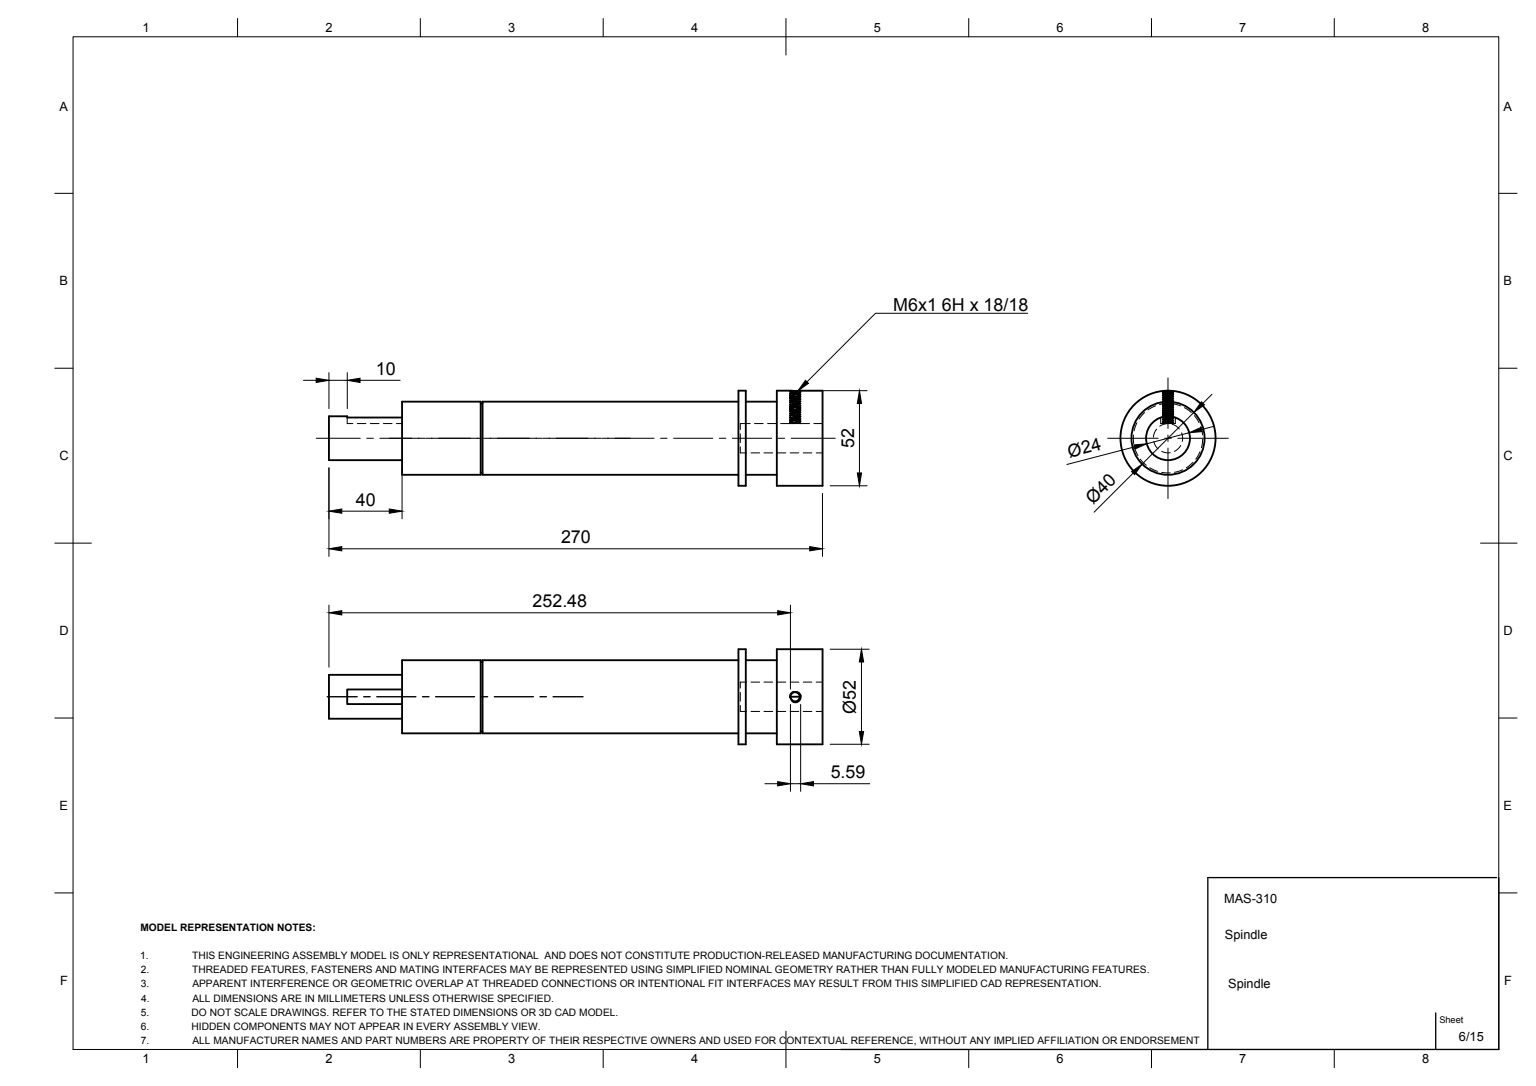
ISO-10303-21;
HEADER;
/* Generated by software containing ST-Developer
 * from STEP Tools, Inc. (www.steptools.com) 
 */

FILE_DESCRIPTION(
/* description */ ('Independent30mm screw-fed quill/spindle unit with16mm straight tool s
ocket, radial set screw, native reusable open ball bearings, retained 
inner/outer race stacks, keyed quill guide and M12x1.75 fine feed. Ext
ernal moving drive and tool not included. Ideal cage orbital links; in
dividual ball spin, force and preload not simulated. No drilling capac
ity, runout, speed, torque, load, life or machine safety rating.'),
/* implementation_level */ '2;1');

FILE_NAME(
/* name */ 'Spindle.step',
/* time_stamp */ '2026-11-08T18:59:42-08:00',
/* author */ (''),
/* organization */ (''),
/* preprocessor_version */ 'ST-DEVELOPER v20.2',
/* originating_system */ 'Autodesk Translation Framework v15.17.0.0',
/* authorisation */ '');

FILE_SCHEMA (('AUTOMOTIVE_DESIGN { 1 0 10303 214 3 1 1 }'));
ENDSEC;

DATA;
#10=MECHANICAL_DESIGN_GEOMETRIC_PRESENTATION_REPRESENTATION('',(#1594),#63898);
#258=B_SPLINE_SURFACE_WITH_KNOTS('',3,3,((#45452,#45453,#45454,#45455,#45456,
#45457,#45458,#45459,#45460,#45461,#45462,#45463,#45464,#45465,#45466,#45467,
#45468,#45469,#45470,#45471,#45472,#45473,#45474,#45475,#45476,#45477,#45478,
#45479,#45480,#45481,#45482,#45483,#45484,#45485,#45486,#45487,#45488,#45489,
#45490,#45491,#45492,#45493,#45494,#45495,#45496,#45497,#45498,#45499,#45500,
#45501,#45502,#45503,#45504,#45505,#45506,#45507,#45508,#45509,#45510,#45511,
#45512,#45513,#45514,#45515,#45516,#45517,#45518,#45519,#45520,#45521,#45522,
#45523,#45524,#45525,#45526,#45527,#45528,#45529,#45530,#45531,#45532,#45533,
#45534,#45535,#45536,#45537,#45538,#45539,#45540,#45541,#45542,#45543,#45544,
#45545,#45546,#45547,#45548,#45549,#45550,#45551,#45552,#45553,#45554,#45555,
#45556,#45557,#45558,#45559,#45560,#45561,#45562,#45563,#45564,#45565,#45566,
#45567,#45568,#45569),(#45570,#45571,#45572,#45573,#45574,#45575,#45576,
#45577,#45578,#45579,#45580,#45581,#45582,#45583,#45584,#45585,#45586,#45587,
#45588,#45589,#45590,#45591,#45592,#45593,#45594,#45595,#45596,#45597,#45598,
#45599,#45600,#45601,#45602,#45603,#45604,#45605,#45606,#45607,#45608,#45609,
#45610,#45611,#45612,#45613,#45614,#45615,#45616,#45617,#45618,#45619,#45620,
#45621,#45622,#45623,#45624,#45625,#45626,#45627,#45628,#45629,#45630,#45631,
#45632,#45633,#45634,#45635,#45636,#45637,#45638,#45639,#45640,#45641,#45642,
#45643,#45644,#45645,#45646,#45647,#45648,#45649,#45650,#45651,#45652,#45653,
#45654,#45655,#45656,#45657,#45658,#45659,#45660,#45661,#45662,#45663,#45664,
#45665,#45666,#45667,#45668,#45669,#45670,#45671,#45672,#45673,#45674,#45675,
#45676,#45677,#45678,#45679,#45680,#45681,#45682,#45683,#45684,#45685,#45686,
#45687),(#45688,#45689,#45690,#45691,#45692,#45693,#45694,#45695,#45696,
#45697,#45698,#45699,#45700,#45701,#45702,#45703,#45704,#45705,#45706,#45707,
#45708,#45709,#45710,#45711,#45712,#45713,#45714,#45715,#45716,#45717,#45718,
#45719,#45720,#45721,#45722,#45723,#45724,#45725,#45726,#45727,#45728,#45729,
#45730,#45731,#45732,#45733,#45734,#45735,#45736,#45737,#45738,#45739,#45740,
#45741,#45742,#45743,#45744,#45745,#45746,#45747,#45748,#45749,#45750,#45751,
#45752,#45753,#45754,#45755,#45756,#45757,#45758,#45759,#45760,#45761,#45762,
#45763,#45764,#45765,#45766,#45767,#45768,#45769,#45770,#45771,#45772,#45773,
#45774,#45775,#45776,#45777,#45778,#45779,#45780,#45781,#45782,#45783,#45784,
#45785,#45786,#45787,#45788,#45789,#45790,#45791,#45792,#45793,#45794,#45795,
#45796,#45797,#45798,#45799,#45800,#45801,#45802,#45803,#45804,#45805),
(#45806,#45807,#45808,#45809,#45810,#45811,#45812,#45813,#45814,#45815,
#45816,#45817,#45818,#45819,#45820,#45821,#45822,#45823,#45824,#45825,#45826,
#45827,#45828,#45829,#45830,#45831,#45832,#45833,#45834,#45835,#45836,#45837,
#45838,#45839,#45840,#45841,#45842,#45843,#45844,#45845,#45846,#45847,#45848,
#45849,#45850,#45851,#45852,#45853,#45854,#45855,#45856,#45857,#45858,#45859,
#45860,#45861,#45862,#45863,#45864,#45865,#45866,#45867,#45868,#45869,#45870,
#45871,#45872,#45873,#45874,#45875,#45876,#45877,#45878,#45879,#45880,#45881,
#45882,#45883,#45884,#45885,#45886,#45887,#45888,#45889,#45890,#45891,#45892,
#45893,#45894,#45895,#45896,#45897,#45898,#45899,#45900,#45901,#45902,#45903,
#45904,#45905,#45906,#45907,#45908,#45909,#45910,#45911,#45912,#45913,#45914,
#45915,#45916,#45917,#45918,#45919,#45920,#45921,#45922,#45923)),
 .UNSPECIFIED.,.F.,.F.,.F.,(4,4),(4,1,1,1,1,1,1,1,1,1,1,1,1,1,1,1,1,1,1,
1,1,1,1,1,1,1,1,1,1,1,1,1,1,1,1,1,1,1,1,1,1,1,1,1,1,1,1,1,1,1,1,1,1,1,1,
1,1,1,1,1,1,1,1,1,1,1,1,1,1,1,1,1,1,1,1,1,1,1,1,1,1,1,1,1,1,1,1,1,1,1,1,
1,1,1,1,1,1,1,1,1,1,1,1,1,1,1,1,1,1,1,1,1,1,1,1,4),(0.,0.0642013499338863),
(12.6240367263184,13.6183778789988,14.6127190316793,15.6070601843597,16.6014013370402,
17.5957424897206,18.590083642401,19.5844247950815,20.5787659477619,21.5731071004423,
22.5674482531228,23.5617894058032,24.5561305584837,25.5504717111641,26.5448128638445,
27.539154016525,28.5334951692054,29.5278363218858,30.5221774745663,31.5165186272467,
32.5108597799272,33.5052009326076,34.499542085288,35.4938832379685,36.4882243906489,
37.4825655433293,38.4769066960098,39.4712478486902,40.4655890013707,41.4599301540511,
42.4542713067315,43.448612459412,44.4429536120924,45.4372947647728,46.4316359174533,
47.4259770701337,48.4203182228142,49.4146593754946,50.409000528175,51.4033416808555,
52.3976828335359,53.3920239862163,54.3863651388968,55.3807062915772,56.3750474442577,
57.3693885969381,58.3637297496185,59.358070902299,60.3524120549794,61.3467532076598,
62.3410943603403,63.3354355130207,64.3297766657012,65.3241178183816,66.318458971062,
67.3128001237425,68.3071412764229,69.3014824291033,70.2958235817838,71.2901647344642,
72.2845058871447,73.2788470398251,74.2731881925055,75.267529345186,76.2618704978664,
77.2562116505468,78.2505528032273,79.2448939559077,80.2392351085882,81.2335762612686,
82.227917413949,83.2222585666295,84.2165997193099,85.2109408719903,86.2052820246708,
87.1996231773512,88.1939643300317,89.1883054827121,90.1826466353925,91.176987788073,
92.1713289407534,93.1656700934338,94.1600112461143,95.1543523987947,96.1486935514752,
97.1430347041556,98.137375856836,99.1317170095165,100.126058162197,101.120399314877,
102.114740467558,103.109081620238,104.103422772919,105.097763925599,106.09210507828,
107.08644623096,108.08078738364,109.075128536321,110.069469689001,111.063810841682,
112.058151994362,113.052493147043,114.046834299723,115.041175452403,116.035516605084,
117.029857757764,118.024198910445,119.018540063125,120.012881215806,121.007222368486,
122.001563521167,122.995904673847,123.990245826527,124.984586979208,125.978928131888,
126.973269284569),.UNSPECIFIED.);
#259=B_SPLINE_SURFACE_WITH_KNOTS('',3,3,((#46071,#46072,#46073,#46074,#46075,
#46076,#46077,#46078,#46079,#46080,#46081,#46082,#46083,#46084,#46085,#46086,
#46087,#46088,#46089,#46090,#46091,#46092,#46093,#46094,#46095,#46096,#46097,
#46098,#46099,#46100,#46101,#46102,#46103,#46104,#46105,#46106,#46107,#46108,
#46109,#46110,#46111,#46112,#46113,#46114,#46115,#46116,#46117,#46118,#46119,
#46120,#46121,#46122,#46123,#46124,#46125,#46126,#46127,#46128,#46129,#46130,
#46131,#46132,#46133,#46134,#46135,#46136,#46137,#46138,#46139,#46140,#46141,
#46142,#46143,#46144,#46145,#46146,#46147,#46148,#46149,#46150,#46151,#46152,
#46153,#46154,#46155,#46156,#46157,#46158,#46159,#46160,#46161,#46162,#46163,
#46164,#46165,#46166,#46167,#46168,#46169,#46170,#46171,#46172,#46173,#46174,
#46175,#46176,#46177,#46178,#46179,#46180,#46181,#46182,#46183,#46184,#46185,
#46186,#46187,#46188),(#46189,#46190,#46191,#46192,#46193,#46194,#46195,
#46196,#46197,#46198,#46199,#46200,#46201,#46202,#46203,#46204,#46205,#46206,
#46207,#46208,#46209,#46210,#46211,#46212,#46213,#46214,#46215,#46216,#46217,
#46218,#46219,#46220,#46221,#46222,#46223,#46224,#46225,#46226,#46227,#46228,
#46229,#46230,#46231,#46232,#46233,#46234,#46235,#46236,#46237,#46238,#46239,
#46240,#46241,#46242,#46243,#46244,#46245,#46246,#46247,#46248,#46249,#46250,
#46251,#46252,#46253,#46254,#46255,#46256,#46257,#46258,#46259,#46260,#46261,
#46262,#46263,#46264,#46265,#46266,#46267,#46268,#46269,#46270,#46271,#46272,
#46273,#46274,#46275,#46276,#46277,#46278,#46279,#46280,#46281,#46282,#46283,
#46284,#46285,#46286,#46287,#46288,#46289,#46290,#46291,#46292,#46293,#46294,
#46295,#46296,#46297,#46298,#46299,#46300,#46301,#46302,#46303,#46304,#46305,
#46306),(#46307,#46308,#46309,#46310,#46311,#46312,#46313,#46314,#46315,
#46316,#46317,#46318,#46319,#46320,#46321,#46322,#46323,#46324,#46325,#46326,
#46327,#46328,#46329,#46330,#46331,#46332,#46333,#46334,#46335,#46336,#46337,
#46338,#46339,#46340,#46341,#46342,#46343,#46344,#46345,#46346,#46347,#46348,
#46349,#46350,#46351,#46352,#46353,#46354,#46355,#46356,#46357,#46358,#46359,
#46360,#46361,#46362,#46363,#46364,#46365,#46366,#46367,#46368,#46369,#46370,
#46371,#46372,#46373,#46374,#46375,#46376,#46377,#46378,#46379,#46380,#46381,
#46382,#46383,#46384,#46385,#46386,#46387,#46388,#46389,#46390,#46391,#46392,
#46393,#46394,#46395,#46396,#46397,#46398,#46399,#46400,#46401,#46402,#46403,
#46404,#46405,#46406,#46407,#46408,#46409,#46410,#46411,#46412,#46413,#46414,
#46415,#46416,#46417,#46418,#46419,#46420,#46421,#46422,#46423,#46424),
(#46425,#46426,#46427,#46428,#46429,#46430,#46431,#46432,#46433,#46434,
#46435,#46436,#46437,#46438,#46439,#46440,#46441,#46442,#46443,#46444,#46445,
#46446,#46447,#46448,#46449,#46450,#46451,#46452,#46453,#46454,#46455,#46456,
#46457,#46458,#46459,#46460,#46461,#46462,#46463,#46464,#46465,#46466,#46467,
#46468,#46469,#46470,#46471,#46472,#46473,#46474,#46475,#46476,#46477,#46478,
#46479,#46480,#46481,#46482,#46483,#46484,#46485,#46486,#46487,#46488,#46489,
#46490,#46491,#46492,#46493,#46494,#46495,#46496,#46497,#46498,#46499,#46500,
#46501,#46502,#46503,#46504,#46505,#46506,#46507,#46508,#46509,#46510,#46511,
#46512,#46513,#46514,#46515,#46516,#46517,#46518,#46519,#46520,#46521,#46522,
#46523,#46524,#46525,#46526,#46527,#46528,#46529,#46530,#46531,#46532,#46533,
#46534,#46535,#46536,#46537,#46538,#46539,#46540,#46541,#46542)),
 .UNSPECIFIED.,.F.,.F.,.F.,(4,4),(4,1,1,1,1,1,1,1,1,1,1,1,1,1,1,1,1,1,1,
1,1,1,1,1,1,1,1,1,1,1,1,1,1,1,1,1,1,1,1,1,1,1,1,1,1,1,1,1,1,1,1,1,1,1,1,
1,1,1,1,1,1,1,1,1,1,1,1,1,1,1,1,1,1,1,1,1,1,1,1,1,1,1,1,1,1,1,1,1,1,1,1,
1,1,1,1,1,1,1,1,1,1,1,1,1,1,1,1,1,1,1,1,1,1,1,1,4),(0.,0.0642013499338863),
(15.4901713080479,16.481671388406,17.4731714687642,18.4646715491223,19.4561716294804,
20.4476717098386,21.4391717901967,22.4306718705548,23.4221719509129,24.4136720312711,
25.4051721116292,26.3966721919873,27.3881722723455,28.3796723527036,29.3711724330617,
30.3626725134198,31.354172593778,32.3456726741361,33.3371727544942,34.3286728348524,
35.3201729152105,36.3116729955686,37.3031730759268,38.2946731562849,39.286173236643,
40.2776733170011,41.2691733973593,42.2606734777174,43.2521735580755,44.2436736384336,
45.2351737187918,46.2266737991499,47.218173879508,48.2096739598662,49.2011740402243,
50.1926741205824,51.1841742009405,52.1756742812987,53.1671743616568,54.1586744420149,
55.1501745223731,56.1416746027312,57.1331746830893,58.1246747634475,59.1161748438056,
60.1076749241637,61.0991750045218,62.09067508488,63.0821751652381,64.0736752455962,
65.0651753259544,66.0566754063125,67.0481754866706,68.0396755670287,69.0311756473869,
70.022675727745,71.0141758081031,72.0056758884613,72.9971759688194,73.9886760491775,
74.9801761295356,75.9716762098938,76.9631762902519,77.95467637061,78.9461764509682,
79.9376765313263,80.9291766116844,81.9206766920425,82.9121767724007,83.9036768527588,
84.8951769331169,85.8866770134751,86.8781770938332,87.8696771741913,88.8611772545494,
89.8526773349076,90.8441774152657,91.8356774956238,92.827177575982,93.8186776563401,
94.8101777366982,95.8016778170563,96.7931778974145,97.7846779777726,98.7761780581307,
99.7676781384889,100.759178218847,101.750678299205,102.742178379563,103.733678459921,
104.72517854028,105.716678620638,106.708178700996,107.699678781354,108.691178861712,
109.68267894207,110.674179022428,111.665679102786,112.657179183145,113.648679263503,
114.640179343861,115.631679424219,116.623179504577,117.614679584935,118.606179665293,
119.597679745651,120.58917982601,121.580679906368,122.572179986726,123.563680067084,
124.555180147442,125.5466802278,126.538180308158,127.529680388516,128.521180468875,
129.512680549233),.UNSPECIFIED.);
#957=B_SPLINE_CURVE_WITH_KNOTS('',3,(#44085,#44086,#44087,#44088),
 .UNSPECIFIED.,.F.,.F.,(4,4),(114.40689867021,115.114280422261),
 .UNSPECIFIED.);
#958=B_SPLINE_CURVE_WITH_KNOTS('',3,(#44093,#44094,#44095,#44096,#44097,
#44098,#44099,#44100,#44101,#44102),.UNSPECIFIED.,.F.,.F.,(4,3,3,4),(-113.097335529233,
-112.13125696422,-111.136915811539,-110.663124627694),.UNSPECIFIED.);
#959=B_SPLINE_CURVE_WITH_KNOTS('',3,(#44107,#44108,#44109,#44110,#44111,
#44112,#44113,#44114,#44115,#44116,#44117,#44118,#44119,#44120,#44121,#44122,
#44123,#44124,#44125,#44126,#44127,#44128,#44129,#44130,#44131),
 .UNSPECIFIED.,.F.,.F.,(4,3,3,3,3,3,3,3,4),(108.12371336303,108.173779859754,
109.165279940112,110.15678002047,111.148280100828,112.139780181187,113.131280261545,
114.122780341903,114.40689867021),.UNSPECIFIED.);
#960=B_SPLINE_CURVE_WITH_KNOTS('',3,(#44132,#44133,#44134,#44135,#44136,
#44137,#44138,#44139,#44140,#44141,#44142,#44143,#44144,#44145,#44146,#44147,
#44148,#44149,#44150,#44151,#44152,#44153),.UNSPECIFIED.,.F.,.F.,(4,3,3,
3,3,3,3,4),(-110.663124627694,-110.142574658859,-109.148233506178,-108.153892353498,
-107.159551200817,-106.165210048137,-105.170868895457,-104.379939320515),
 .UNSPECIFIED.);
#961=B_SPLINE_CURVE_WITH_KNOTS('',3,(#44158,#44159,#44160,#44161,#44162,
#44163,#44164,#44165,#44166,#44167,#44168,#44169,#44170,#44171,#44172,#44173,
#44174,#44175,#44176,#44177,#44178,#44179),.UNSPECIFIED.,.F.,.F.,(4,3,3,
3,3,3,3,4),(101.84052805585,102.224779377605,103.216279457963,104.207779538322,
105.19927961868,106.190779699038,107.182279779396,108.12371336303),
 .UNSPECIFIED.);
#962=B_SPLINE_CURVE_WITH_KNOTS('',3,(#44180,#44181,#44182,#44183,#44184,
#44185,#44186,#44187,#44188,#44189,#44190,#44191,#44192,#44193,#44194,#44195,
#44196,#44197,#44198,#44199,#44200,#44201,#44202,#44203,#44204),
 .UNSPECIFIED.,.F.,.F.,(4,3,3,3,3,3,3,3,4),(-104.379939320515,-104.176527742776,
-103.182186590096,-102.187845437415,-101.193504284735,-100.199163132054,
-99.204821979374,-98.2104808266935,-98.096754013335),.UNSPECIFIED.);
#963=B_SPLINE_CURVE_WITH_KNOTS('',3,(#44209,#44210,#44211,#44212,#44213,
#44214,#44215,#44216,#44217,#44218,#44219,#44220,#44221,#44222,#44223,#44224,
#44225,#44226,#44227,#44228,#44229,#44230),.UNSPECIFIED.,.F.,.F.,(4,3,3,
3,3,3,3,4),(95.5573427486709,96.2757788954565,97.2672789758147,98.2587790561728,
99.2502791365309,100.241779216889,101.233279297247,101.84052805585),
 .UNSPECIFIED.);
#964=B_SPLINE_CURVE_WITH_KNOTS('',3,(#44231,#44232,#44233,#44234,#44235,
#44236,#44237,#44238,#44239,#44240,#44241,#44242,#44243,#44244,#44245,#44246,
#44247,#44248,#44249,#44250,#44251,#44252),.UNSPECIFIED.,.F.,.F.,(4,3,3,
3,3,3,3,4),(-98.096754013335,-97.2161396740131,-96.2217985213327,-95.2274573686523,
-94.2331162159718,-93.2387750632914,-92.2444339106109,-91.8135687061554),
 .UNSPECIFIED.);
#965=B_SPLINE_CURVE_WITH_KNOTS('',3,(#44257,#44258,#44259,#44260,#44261,
#44262,#44263,#44264,#44265,#44266,#44267,#44268,#44269,#44270,#44271,#44272,
#44273,#44274,#44275,#44276,#44277,#44278,#44279,#44280,#44281),
 .UNSPECIFIED.,.F.,.F.,(4,3,3,3,3,3,3,3,4),(89.2741574414913,89.3352783329496,
90.3267784133077,91.3182784936659,92.309778574024,93.3012786543821,94.2927787347403,
95.2842788150984,95.5573427486709),.UNSPECIFIED.);
#966=B_SPLINE_CURVE_WITH_KNOTS('',3,(#44282,#44283,#44284,#44285,#44286,
#44287,#44288,#44289,#44290,#44291,#44292,#44293,#44294,#44295,#44296,#44297,
#44298,#44299,#44300,#44301,#44302,#44303),.UNSPECIFIED.,.F.,.F.,(4,3,3,
3,3,3,3,4),(-91.8135687061554,-91.2500927579305,-90.2557516052501,-89.2614104525696,
-88.2670692998892,-87.2727281472088,-86.2783869945283,-85.5303833989758),
 .UNSPECIFIED.);
#967=B_SPLINE_CURVE_WITH_KNOTS('',3,(#44308,#44309,#44310,#44311,#44312,
#44313,#44314,#44315,#44316,#44317,#44318,#44319,#44320,#44321,#44322,#44323,
#44324,#44325,#44326,#44327,#44328,#44329),.UNSPECIFIED.,.F.,.F.,(4,3,3,
3,3,3,3,4),(82.9909721343117,83.3862778508009,84.377777931159,85.3692780115171,
86.3607780918753,87.3522781722334,88.3437782525915,89.2741574414913),
 .UNSPECIFIED.);
#968=B_SPLINE_CURVE_WITH_KNOTS('',3,(#44330,#44331,#44332,#44333,#44334,
#44335,#44336,#44337,#44338,#44339,#44340,#44341,#44342,#44343,#44344,#44345,
#44346,#44347,#44348,#44349,#44350,#44351,#44352,#44353,#44354),
 .UNSPECIFIED.,.F.,.F.,(4,3,3,3,3,3,3,3,4),(-85.5303833989758,-85.2840458418479,
-84.2897046891674,-83.295363536487,-82.3010223838066,-81.3066812311261,
-80.3123400784457,-79.3179989257652,-79.2471980917962),.UNSPECIFIED.);
#969=B_SPLINE_CURVE_WITH_KNOTS('',3,(#44359,#44360,#44361,#44362,#44363,
#44364,#44365,#44366,#44367,#44368,#44369,#44370,#44371,#44372,#44373,#44374,
#44375,#44376,#44377,#44378,#44379,#44380),.UNSPECIFIED.,.F.,.F.,(4,3,3,
3,3,3,3,4),(76.7077868271321,77.4372773686521,78.4287774490102,79.4202775293683,
80.4117776097265,81.4032776900846,82.3947777704427,82.9909721343117),
 .UNSPECIFIED.);
#970=B_SPLINE_CURVE_WITH_KNOTS('',3,(#44381,#44382,#44383,#44384,#44385,
#44386,#44387,#44388,#44389,#44390,#44391,#44392,#44393,#44394,#44395,#44396,
#44397,#44398,#44399,#44400,#44401,#44402),.UNSPECIFIED.,.F.,.F.,(4,3,3,
3,3,3,3,4),(-79.2471980917962,-78.3236577730848,-77.3293166204044,-76.3349754677239,
-75.3406343150435,-74.3462931623631,-73.3519520096826,-72.9640127846166),
 .UNSPECIFIED.);
#971=B_SPLINE_CURVE_WITH_KNOTS('',3,(#44407,#44408,#44409,#44410,#44411,
#44412,#44413,#44414,#44415,#44416,#44417,#44418,#44419,#44420,#44421,#44422,
#44423,#44424,#44425,#44426,#44427,#44428,#44429,#44430,#44431),
 .UNSPECIFIED.,.F.,.F.,(4,3,3,3,3,3,3,3,4),(70.4246015199525,70.4967768061452,
71.4882768865033,72.4797769668614,73.4712770472196,74.4627771275777,75.4542772079358,
76.445777288294,76.7077868271321),.UNSPECIFIED.);
#972=B_SPLINE_CURVE_WITH_KNOTS('',3,(#44432,#44433,#44434,#44435,#44436,
#44437,#44438,#44439,#44440,#44441,#44442,#44443,#44444,#44445,#44446,#44447,
#44448,#44449,#44450,#44451,#44452,#44453),.UNSPECIFIED.,.F.,.F.,(4,3,3,
3,3,3,3,4),(-72.9640127846166,-72.3576108570022,-71.3632697043217,-70.3689285516413,
-69.3745873989609,-68.3802462462804,-67.3859050936,-66.680827477437),
 .UNSPECIFIED.);
#973=B_SPLINE_CURVE_WITH_KNOTS('',3,(#44458,#44459,#44460,#44461,#44462,
#44463,#44464,#44465,#44466,#44467,#44468,#44469,#44470,#44471,#44472,#44473,
#44474,#44475,#44476,#44477,#44478,#44479),.UNSPECIFIED.,.F.,.F.,(4,3,3,
3,3,3,3,4),(64.1414162127729,64.5477763239964,65.5392764043545,66.5307764847127,
67.5222765650708,68.5137766454289,69.5052767257871,70.4246015199525),
 .UNSPECIFIED.);
#974=B_SPLINE_CURVE_WITH_KNOTS('',3,(#44480,#44481,#44482,#44483,#44484,
#44485,#44486,#44487,#44488,#44489,#44490,#44491,#44492,#44493,#44494,#44495,
#44496,#44497,#44498,#44499,#44500,#44501,#44502,#44503,#44504),
 .UNSPECIFIED.,.F.,.F.,(4,3,3,3,3,3,3,3,4),(-66.680827477437,-66.3915639409195,
-65.3972227882391,-64.4028816355587,-63.4085404828782,-62.4141993301978,
-61.4198581775174,-60.4255170248369,-60.3976421702574),.UNSPECIFIED.);
#975=B_SPLINE_CURVE_WITH_KNOTS('',3,(#44509,#44510,#44511,#44512,#44513,
#44514,#44515,#44516,#44517,#44518,#44519,#44520,#44521,#44522,#44523,#44524,
#44525,#44526,#44527,#44528,#44529,#44530),.UNSPECIFIED.,.F.,.F.,(4,3,3,
3,3,3,3,4),(57.8582309055933,58.5987758418476,59.5902759222058,60.5817760025639,
61.573276082922,62.5647761632802,63.5562762436383,64.1414162127729),
 .UNSPECIFIED.);
#976=B_SPLINE_CURVE_WITH_KNOTS('',3,(#44531,#44532,#44533,#44534,#44535,
#44536,#44537,#44538,#44539,#44540,#44541,#44542,#44543,#44544,#44545,#44546,
#44547,#44548,#44549,#44550,#44551,#44552),.UNSPECIFIED.,.F.,.F.,(4,3,3,
3,3,3,3,4),(-60.3976421702574,-59.4311758721565,-58.4368347194761,-57.4424935667956,
-56.4481524141152,-55.4538112614347,-54.4594701087543,-54.1144568630778),
 .UNSPECIFIED.);
#977=B_SPLINE_CURVE_WITH_KNOTS('',3,(#44557,#44558,#44559,#44560,#44561,
#44562,#44563,#44564,#44565,#44566,#44567,#44568,#44569,#44570,#44571,#44572,
#44573,#44574,#44575,#44576,#44577,#44578,#44579,#44580,#44581),
 .UNSPECIFIED.,.F.,.F.,(4,3,3,3,3,3,3,3,4),(51.5750455984137,51.6582752793407,
52.6497753596989,53.641275440057,54.6327755204151,55.6242756007733,56.6157756811314,
57.6072757614895,57.8582309055933),.UNSPECIFIED.);
#978=B_SPLINE_CURVE_WITH_KNOTS('',3,(#44582,#44583,#44584,#44585,#44586,
#44587,#44588,#44589,#44590,#44591,#44592,#44593,#44594,#44595,#44596,#44597,
#44598,#44599,#44600,#44601,#44602,#44603),.UNSPECIFIED.,.F.,.F.,(4,3,3,
3,3,3,3,4),(-54.1144568630778,-53.4651289560739,-52.4707878033934,-51.476446650713,
-50.4821054980325,-49.4877643453521,-48.4934231926717,-47.8312715558982),
 .UNSPECIFIED.);
#979=B_SPLINE_CURVE_WITH_KNOTS('',3,(#44608,#44609,#44610,#44611,#44612,
#44613,#44614,#44615,#44616,#44617,#44618,#44619,#44620,#44621,#44622,#44623,
#44624,#44625,#44626,#44627,#44628,#44629),.UNSPECIFIED.,.F.,.F.,(4,3,3,
3,3,3,3,4),(45.2918602912341,45.709274797192,46.7007748775501,47.6922749579082,
48.6837750382664,49.6752751186245,50.6667751989826,51.5750455984137),
 .UNSPECIFIED.);
#980=B_SPLINE_CURVE_WITH_KNOTS('',3,(#44630,#44631,#44632,#44633,#44634,
#44635,#44636,#44637,#44638,#44639,#44640,#44641,#44642,#44643,#44644,#44645,
#44646,#44647,#44648,#44649,#44650,#44651),.UNSPECIFIED.,.F.,.F.,(4,3,3,
3,3,3,3,4),(-47.8312715558982,-47.4990820399912,-46.5047408873108,-45.5103997346304,
-44.5160585819499,-43.5217174292695,-42.5273762765891,-41.5480862487186),
 .UNSPECIFIED.);
#981=B_SPLINE_CURVE_WITH_KNOTS('',3,(#44656,#44657,#44658,#44659,#44660,
#44661,#44662,#44663,#44664,#44665,#44666,#44667,#44668,#44669,#44670,#44671,
#44672,#44673,#44674,#44675,#44676,#44677),.UNSPECIFIED.,.F.,.F.,(4,3,3,
3,3,3,3,4),(39.0086749840545,39.7602743150432,40.7517743954013,41.7432744757595,
42.7347745561176,43.7262746364757,44.7177747168338,45.2918602912341),
 .UNSPECIFIED.);
#982=B_SPLINE_CURVE_WITH_KNOTS('',3,(#44678,#44679,#44680,#44681,#44682,
#44683,#44684,#44685,#44686,#44687,#44688,#44689,#44690,#44691,#44692,#44693,
#44694,#44695,#44696,#44697,#44698,#44699,#44700,#44701,#44702),
 .UNSPECIFIED.,.F.,.F.,(4,3,3,3,3,3,3,3,4),(-41.5480862487186,-41.5330351239086,
-40.5386939712282,-39.5443528185478,-38.5500116658673,-37.5556705131869,
-36.5613293605064,-35.566988207826,-35.264900941539),.UNSPECIFIED.);
#983=B_SPLINE_CURVE_WITH_KNOTS('',3,(#44707,#44708,#44709,#44710,#44711,
#44712,#44713,#44714,#44715,#44716,#44717,#44718,#44719,#44720,#44721,#44722,
#44723,#44724,#44725,#44726,#44727,#44728,#44729,#44730,#44731),
 .UNSPECIFIED.,.F.,.F.,(4,3,3,3,3,3,3,3,4),(32.725489676875,32.8197737525363,
33.8112738328944,34.8027739132525,35.7942739936107,36.7857740739688,37.7772741543269,
38.7687742346851,39.0086749840545),.UNSPECIFIED.);
#984=B_SPLINE_CURVE_WITH_KNOTS('',3,(#44732,#44733,#44734,#44735,#44736,
#44737,#44738,#44739,#44740,#44741,#44742,#44743,#44744,#44745,#44746,#44747,
#44748,#44749,#44750,#44751,#44752,#44753),.UNSPECIFIED.,.F.,.F.,(4,3,3,
3,3,3,3,4),(-35.264900941539,-34.5726470551456,-33.5783059024651,-32.5839647497847,
-31.5896235971042,-30.5952824444238,-29.6009412917434,-28.9817156343595),
 .UNSPECIFIED.);
#985=B_SPLINE_CURVE_WITH_KNOTS('',3,(#44758,#44759,#44760,#44761,#44762,
#44763,#44764,#44765,#44766,#44767,#44768,#44769,#44770,#44771,#44772,#44773,
#44774,#44775,#44776,#44777,#44778,#44779),.UNSPECIFIED.,.F.,.F.,(4,3,3,
3,3,3,3,4),(26.4423043696954,26.8707732703875,27.8622733507456,28.8537734311038,
29.8452735114619,30.83677359182,31.8282736721782,32.725489676875),
 .UNSPECIFIED.);
#986=B_SPLINE_CURVE_WITH_KNOTS('',3,(#44780,#44781,#44782,#44783,#44784,
#44785,#44786,#44787,#44788,#44789,#44790,#44791,#44792,#44793,#44794,#44795,
#44796,#44797,#44798,#44799,#44800,#44801),.UNSPECIFIED.,.F.,.F.,(4,3,3,
3,3,3,3,4),(-28.9817156343595,-28.6066001390629,-27.6122589863825,-26.6179178337021,
-25.6235766810216,-24.6292355283412,-23.6348943756607,-22.6985303271799),
 .UNSPECIFIED.);
#987=B_SPLINE_CURVE_WITH_KNOTS('',3,(#44806,#44807,#44808,#44809,#44810,
#44811,#44812,#44813,#44814,#44815,#44816,#44817,#44818,#44819,#44820,#44821,
#44822,#44823,#44824,#44825,#44826,#44827),.UNSPECIFIED.,.F.,.F.,(4,3,3,
3,3,3,3,4),(20.1591190625158,20.9217727882387,21.9132728685969,22.904772948955,
23.8962730293131,24.8877731096713,25.8792731900294,26.4423043696954),
 .UNSPECIFIED.);
#988=B_SPLINE_CURVE_WITH_KNOTS('',3,(#44828,#44829,#44830,#44831,#44832,
#44833,#44834,#44835,#44836,#44837,#44838,#44839,#44840,#44841,#44842,#44843,
#44844,#44845,#44846,#44847,#44848,#44849,#44850,#44851,#44852),
 .UNSPECIFIED.,.F.,.F.,(4,3,3,3,3,3,3,3,4),(-22.6985303271799,-22.6405532229803,
-21.6462120702999,-20.6518709176194,-19.657529764939,-18.6631886122585,
-17.6688474595781,-16.6745063068977,-16.4153450200003),.UNSPECIFIED.);
#989=B_SPLINE_CURVE_WITH_KNOTS('',3,(#44857,#44858,#44859,#44860,#44861,
#44862,#44863,#44864,#44865,#44866,#44867,#44868,#44869,#44870,#44871,#44872,
#44873,#44874,#44875,#44876,#44877,#44878,#44879,#44880,#44881),
 .UNSPECIFIED.,.F.,.F.,(4,3,3,3,3,3,3,3,4),(13.8759337553362,13.9812722257318,
14.97277230609,15.9642723864481,16.9557724668062,17.9472725471644,18.9387726275225,
19.9302727078806,20.1591190625158),.UNSPECIFIED.);
#990=B_SPLINE_CURVE_WITH_KNOTS('',3,(#44882,#44883,#44884,#44885,#44886,
#44887,#44888,#44889,#44890,#44891,#44892,#44893,#44894,#44895,#44896,#44897,
#44898,#44899,#44900,#44901,#44902,#44903),.UNSPECIFIED.,.F.,.F.,(4,3,3,
3,3,3,3,4),(-16.4153450200003,-15.6801651542172,-14.6858240015368,-13.6914828488564,
-12.6971416961759,-11.7028005434955,-10.708459390815,-10.1321597128207),
 .UNSPECIFIED.);
#991=B_SPLINE_CURVE_WITH_KNOTS('',3,(#44909,#44910,#44911,#44912,#44913,
#44914,#44915,#44916,#44917,#44918,#44919,#44920,#44921),.UNSPECIFIED.,
 .F.,.F.,(4,3,3,3,4),(-3.84897440564112,-3.74807132205199,-2.75373016937155,
-1.75938901669111,-0.765047864010683),.UNSPECIFIED.);
#992=B_SPLINE_CURVE_WITH_KNOTS('',3,(#44923,#44924,#44925,#44926,#44927,
#44928,#44929,#44930,#44931,#44932,#44933,#44934,#44935,#44936,#44937,#44938),
 .UNSPECIFIED.,.F.,.F.,(4,2,2,2,2,2,2,4),(0.232635770676731,0.284684236160853,
0.379578792383291,0.47447334860573,0.569367904828168,0.664262744797375,
0.759157584766583,0.773538308589687),.UNSPECIFIED.);
#993=B_SPLINE_CURVE_WITH_KNOTS('',3,(#44939,#44940,#44941,#44942,#44943,
#44944,#44945,#44946,#44947,#44948,#44949,#44950,#44951,#44952,#44953,#44954,
#44955,#44956,#44957),.UNSPECIFIED.,.F.,.F.,(4,3,3,3,3,3,4),(2.26925352322945,
3.07477134179243,4.06627142215055,5.05777150250868,6.04927158286681,7.04077166322494,
7.59274844815659),.UNSPECIFIED.);
#994=B_SPLINE_CURVE_WITH_KNOTS('',3,(#44963,#44964,#44965,#44966,#44967,
#44968,#44969,#44970),.UNSPECIFIED.,.F.,.F.,(4,1,1,1,1,4),(122.522113490002,
122.995904673847,123.990245826527,124.984586979208,125.978928131888,126.973269284569),
 .UNSPECIFIED.);
#995=B_SPLINE_CURVE_WITH_KNOTS('',3,(#44975,#44976,#44977,#44978,#44979,
#44980,#44981,#44982,#44983),.UNSPECIFIED.,.F.,.F.,(4,1,1,1,1,1,4),(122.522113490002,
122.572179986726,123.563680067084,124.555180147442,125.5466802278,126.538180308158,
127.495735656204),.UNSPECIFIED.);
#996=B_SPLINE_CURVE_WITH_KNOTS('',3,(#44988,#44989,#44990,#44991,#44992,
#44993,#44994,#44995,#44996,#44997),.UNSPECIFIED.,.F.,.F.,(4,1,1,1,1,1,
1,4),(116.238928182822,117.029857757764,118.024198910445,119.018540063125,
120.012881215806,121.007222368486,122.001563521167,122.522113490002),
 .UNSPECIFIED.);
#997=B_SPLINE_CURVE_WITH_KNOTS('',3,(#44998,#44999,#45000,#45001,#45002,
#45003,#45004,#45005,#45006,#45007),.UNSPECIFIED.,.F.,.F.,(4,1,1,1,1,1,
1,4),(116.238928182822,116.623179504577,117.614679584935,118.606179665293,
119.597679745651,120.58917982601,121.580679906368,122.522113490002),
 .UNSPECIFIED.);
#998=B_SPLINE_CURVE_WITH_KNOTS('',3,(#45012,#45013,#45014,#45015,#45016,
#45017,#45018,#45019,#45020,#45021,#45022),.UNSPECIFIED.,.F.,.F.,(4,1,1,
1,1,1,1,1,4),(109.955742875643,110.069469689001,111.063810841682,112.058151994362,
113.052493147043,114.046834299723,115.041175452403,116.035516605084,116.238928182822),
 .UNSPECIFIED.);
#999=B_SPLINE_CURVE_WITH_KNOTS('',3,(#45023,#45024,#45025,#45026,#45027,
#45028,#45029,#45030,#45031,#45032),.UNSPECIFIED.,.F.,.F.,(4,1,1,1,1,1,
1,4),(109.955742875643,110.674179022428,111.665679102786,112.657179183145,
113.648679263503,114.640179343861,115.631679424219,116.238928182822),
 .UNSPECIFIED.);
#1000=B_SPLINE_CURVE_WITH_KNOTS('',3,(#45037,#45038,#45039,#45040,#45041,
#45042,#45043,#45044,#45045,#45046),.UNSPECIFIED.,.F.,.F.,(4,1,1,1,1,1,
1,4),(103.672557568463,104.103422772919,105.097763925599,106.09210507828,
107.08644623096,108.08078738364,109.075128536321,109.955742875643),
 .UNSPECIFIED.);
#1001=B_SPLINE_CURVE_WITH_KNOTS('',3,(#45047,#45048,#45049,#45050,#45051,
#45052,#45053,#45054,#45055,#45056,#45057),.UNSPECIFIED.,.F.,.F.,(4,1,1,
1,1,1,1,1,4),(103.672557568463,103.733678459921,104.72517854028,105.716678620638,
106.708178700996,107.699678781354,108.691178861712,109.68267894207,109.955742875643),
 .UNSPECIFIED.);
#1002=B_SPLINE_CURVE_WITH_KNOTS('',3,(#45062,#45063,#45064,#45065,#45066,
#45067,#45068,#45069,#45070,#45071),.UNSPECIFIED.,.F.,.F.,(4,1,1,1,1,1,
1,4),(97.3893722612835,98.137375856836,99.1317170095165,100.126058162197,
101.120399314877,102.114740467558,103.109081620238,103.672557568463),
 .UNSPECIFIED.);
#1003=B_SPLINE_CURVE_WITH_KNOTS('',3,(#45072,#45073,#45074,#45075,#45076,
#45077,#45078,#45079,#45080,#45081),.UNSPECIFIED.,.F.,.F.,(4,1,1,1,1,1,
1,4),(97.3893722612835,97.7846779777726,98.7761780581307,99.7676781384889,
100.759178218847,101.750678299205,102.742178379563,103.672557568463),
 .UNSPECIFIED.);
#1004=B_SPLINE_CURVE_WITH_KNOTS('',3,(#45086,#45087,#45088,#45089,#45090,
#45091,#45092,#45093,#45094,#45095,#45096),.UNSPECIFIED.,.F.,.F.,(4,1,1,
1,1,1,1,1,4),(91.1061869541039,91.176987788073,92.1713289407534,93.1656700934338,
94.1600112461143,95.1543523987947,96.1486935514752,97.1430347041556,97.3893722612835),
 .UNSPECIFIED.);
#1005=B_SPLINE_CURVE_WITH_KNOTS('',3,(#45097,#45098,#45099,#45100,#45101,
#45102,#45103,#45104,#45105,#45106),.UNSPECIFIED.,.F.,.F.,(4,1,1,1,1,1,
1,4),(91.1061869541039,91.8356774956238,92.827177575982,93.8186776563401,
94.8101777366982,95.8016778170563,96.7931778974145,97.3893722612835),
 .UNSPECIFIED.);
#1006=B_SPLINE_CURVE_WITH_KNOTS('',3,(#45111,#45112,#45113,#45114,#45115,
#45116,#45117,#45118,#45119,#45120),.UNSPECIFIED.,.F.,.F.,(4,1,1,1,1,1,
1,4),(84.8230016469244,85.2109408719903,86.2052820246708,87.1996231773512,
88.1939643300317,89.1883054827121,90.1826466353925,91.1061869541039),
 .UNSPECIFIED.);
#1007=B_SPLINE_CURVE_WITH_KNOTS('',3,(#45121,#45122,#45123,#45124,#45125,
#45126,#45127,#45128,#45129,#45130,#45131),.UNSPECIFIED.,.F.,.F.,(4,1,1,
1,1,1,1,1,4),(84.8230016469244,84.8951769331169,85.8866770134751,86.8781770938332,
87.8696771741913,88.8611772545494,89.8526773349076,90.8441774152657,91.1061869541039),
 .UNSPECIFIED.);
#1008=B_SPLINE_CURVE_WITH_KNOTS('',3,(#45136,#45137,#45138,#45139,#45140,
#45141,#45142,#45143,#45144,#45145),.UNSPECIFIED.,.F.,.F.,(4,1,1,1,1,1,
1,4),(78.5398163397448,79.2448939559077,80.2392351085882,81.2335762612686,
82.227917413949,83.2222585666295,84.2165997193099,84.8230016469244),
 .UNSPECIFIED.);
#1009=B_SPLINE_CURVE_WITH_KNOTS('',3,(#45146,#45147,#45148,#45149,#45150,
#45151,#45152,#45153,#45154,#45155),.UNSPECIFIED.,.F.,.F.,(4,1,1,1,1,1,
1,4),(78.5398163397448,78.9461764509682,79.9376765313263,80.9291766116844,
81.9206766920425,82.9121767724007,83.9036768527588,84.8230016469244),
 .UNSPECIFIED.);
#1010=B_SPLINE_CURVE_WITH_KNOTS('',3,(#45160,#45161,#45162,#45163,#45164,
#45165,#45166,#45167,#45168,#45169,#45170),.UNSPECIFIED.,.F.,.F.,(4,1,1,
1,1,1,1,1,4),(72.2566310325652,72.2845058871447,73.2788470398251,74.2731881925055,
75.267529345186,76.2618704978664,77.2562116505468,78.2505528032273,78.5398163397448),
 .UNSPECIFIED.);
#1011=B_SPLINE_CURVE_WITH_KNOTS('',3,(#45171,#45172,#45173,#45174,#45175,
#45176,#45177,#45178,#45179,#45180),.UNSPECIFIED.,.F.,.F.,(4,1,1,1,1,1,
1,4),(72.2566310325652,72.9971759688194,73.9886760491775,74.9801761295356,
75.9716762098938,76.9631762902519,77.95467637061,78.5398163397448),
 .UNSPECIFIED.);
#1012=B_SPLINE_CURVE_WITH_KNOTS('',3,(#45185,#45186,#45187,#45188,#45189,
#45190,#45191,#45192,#45193,#45194),.UNSPECIFIED.,.F.,.F.,(4,1,1,1,1,1,
1,4),(65.9734457253856,66.318458971062,67.3128001237425,68.3071412764229,
69.3014824291033,70.2958235817838,71.2901647344642,72.2566310325652),
 .UNSPECIFIED.);
#1013=B_SPLINE_CURVE_WITH_KNOTS('',3,(#45195,#45196,#45197,#45198,#45199,
#45200,#45201,#45202,#45203,#45204,#45205),.UNSPECIFIED.,.F.,.F.,(4,1,1,
1,1,1,1,1,4),(65.9734457253856,66.0566754063125,67.0481754866706,68.0396755670287,
69.0311756473869,70.022675727745,71.0141758081031,72.0056758884613,72.2566310325652),
 .UNSPECIFIED.);
#1014=B_SPLINE_CURVE_WITH_KNOTS('',3,(#45210,#45211,#45212,#45213,#45214,
#45215,#45216,#45217,#45218,#45219),.UNSPECIFIED.,.F.,.F.,(4,1,1,1,1,1,
1,4),(59.690260418206,60.3524120549794,61.3467532076598,62.3410943603403,
63.3354355130207,64.3297766657012,65.3241178183816,65.9734457253856),
 .UNSPECIFIED.);
#1015=B_SPLINE_CURVE_WITH_KNOTS('',3,(#45220,#45221,#45222,#45223,#45224,
#45225,#45226,#45227,#45228,#45229),.UNSPECIFIED.,.F.,.F.,(4,1,1,1,1,1,
1,4),(59.690260418206,60.1076749241637,61.0991750045218,62.09067508488,
63.0821751652381,64.0736752455962,65.0651753259544,65.9734457253856),
 .UNSPECIFIED.);
#1016=B_SPLINE_CURVE_WITH_KNOTS('',3,(#45234,#45235,#45236,#45237,#45238,
#45239,#45240,#45241,#45242,#45243),.UNSPECIFIED.,.F.,.F.,(4,1,1,1,1,1,
1,4),(53.4070751110264,54.3863651388968,55.3807062915772,56.3750474442577,
57.3693885969381,58.3637297496185,59.358070902299,59.690260418206),
 .UNSPECIFIED.);
#1017=B_SPLINE_CURVE_WITH_KNOTS('',3,(#45244,#45245,#45246,#45247,#45248,
#45249,#45250,#45251,#45252,#45253),.UNSPECIFIED.,.F.,.F.,(4,1,1,1,1,1,
1,4),(53.4070751110264,54.1586744420149,55.1501745223731,56.1416746027312,
57.1331746830893,58.1246747634475,59.1161748438056,59.690260418206),
 .UNSPECIFIED.);
#1018=B_SPLINE_CURVE_WITH_KNOTS('',3,(#45258,#45259,#45260,#45261,#45262,
#45263,#45264,#45265,#45266,#45267,#45268),.UNSPECIFIED.,.F.,.F.,(4,1,1,
1,1,1,1,1,4),(47.1238898038468,47.4259770701337,48.4203182228142,49.4146593754946,
50.409000528175,51.4033416808555,52.3976828335359,53.3920239862163,53.4070751110264),
 .UNSPECIFIED.);
#1019=B_SPLINE_CURVE_WITH_KNOTS('',3,(#45269,#45270,#45271,#45272,#45273,
#45274,#45275,#45276,#45277,#45278,#45279),.UNSPECIFIED.,.F.,.F.,(4,1,1,
1,1,1,1,1,4),(47.1238898038468,47.218173879508,48.2096739598662,49.2011740402243,
50.1926741205824,51.1841742009405,52.1756742812987,53.1671743616568,53.4070751110264),
 .UNSPECIFIED.);
#1020=B_SPLINE_CURVE_WITH_KNOTS('',3,(#45284,#45285,#45286,#45287,#45288,
#45289,#45290,#45291,#45292,#45293),.UNSPECIFIED.,.F.,.F.,(4,1,1,1,1,1,
1,4),(40.8407044966672,41.4599301540511,42.4542713067315,43.448612459412,
44.4429536120924,45.4372947647728,46.4316359174533,47.1238898038468),
 .UNSPECIFIED.);
#1021=B_SPLINE_CURVE_WITH_KNOTS('',3,(#45294,#45295,#45296,#45297,#45298,
#45299,#45300,#45301,#45302,#45303),.UNSPECIFIED.,.F.,.F.,(4,1,1,1,1,1,
1,4),(40.8407044966672,41.2691733973593,42.2606734777174,43.2521735580755,
44.2436736384336,45.2351737187918,46.2266737991499,47.1238898038468),
 .UNSPECIFIED.);
#1022=B_SPLINE_CURVE_WITH_KNOTS('',3,(#45308,#45309,#45310,#45311,#45312,
#45313,#45314,#45315,#45316,#45317),.UNSPECIFIED.,.F.,.F.,(4,1,1,1,1,1,
1,4),(34.5575191894876,35.4938832379685,36.4882243906489,37.4825655433293,
38.4769066960098,39.4712478486902,40.4655890013707,40.8407044966672),
 .UNSPECIFIED.);
#1023=B_SPLINE_CURVE_WITH_KNOTS('',3,(#45318,#45319,#45320,#45321,#45322,
#45323,#45324,#45325,#45326,#45327),.UNSPECIFIED.,.F.,.F.,(4,1,1,1,1,1,
1,4),(34.5575191894876,35.3201729152105,36.3116729955686,37.3031730759268,
38.2946731562849,39.286173236643,40.2776733170011,40.8407044966672),
 .UNSPECIFIED.);
#1024=B_SPLINE_CURVE_WITH_KNOTS('',3,(#45332,#45333,#45334,#45335,#45336,
#45337,#45338,#45339,#45340,#45341,#45342),.UNSPECIFIED.,.F.,.F.,(4,1,1,
1,1,1,1,1,4),(28.274333882308,28.5334951692054,29.5278363218858,30.5221774745663,
31.5165186272467,32.5108597799272,33.5052009326076,34.499542085288,34.5575191894876),
 .UNSPECIFIED.);
#1025=B_SPLINE_CURVE_WITH_KNOTS('',3,(#45343,#45344,#45345,#45346,#45347,
#45348,#45349,#45350,#45351,#45352,#45353),.UNSPECIFIED.,.F.,.F.,(4,1,1,
1,1,1,1,1,4),(28.274333882308,28.3796723527036,29.3711724330617,30.3626725134198,
31.354172593778,32.3456726741361,33.3371727544942,34.3286728348524,34.5575191894876),
 .UNSPECIFIED.);
#1026=B_SPLINE_CURVE_WITH_KNOTS('',3,(#45358,#45359,#45360,#45361,#45362,
#45363,#45364,#45365,#45366,#45367),.UNSPECIFIED.,.F.,.F.,(4,1,1,1,1,1,
1,4),(21.9911485751284,22.5674482531228,23.5617894058032,24.5561305584837,
25.5504717111641,26.5448128638445,27.539154016525,28.274333882308),
 .UNSPECIFIED.);
#1027=B_SPLINE_CURVE_WITH_KNOTS('',3,(#45368,#45369,#45370,#45371,#45372,
#45373,#45374,#45375,#45376,#45377),.UNSPECIFIED.,.F.,.F.,(4,1,1,1,1,1,
1,4),(21.9911485751284,22.4306718705548,23.4221719509129,24.4136720312711,
25.4051721116292,26.3966721919873,27.3881722723455,28.274333882308),
 .UNSPECIFIED.);
#1028=B_SPLINE_CURVE_WITH_KNOTS('',3,(#45383,#45384,#45385,#45386),
 .UNSPECIFIED.,.F.,.F.,(4,4),(15.4901713080479,15.7079632679489),
 .UNSPECIFIED.);
#1029=B_SPLINE_CURVE_WITH_KNOTS('',3,(#45388,#45389,#45390,#45391,#45392,
#45393,#45394,#45395,#45396,#45397),.UNSPECIFIED.,.F.,.F.,(4,2,2,2,4),(1.39069260388053,
1.50658326762018,1.62247393135982,1.73836536826693,1.78923484994644),
 .UNSPECIFIED.);
#1030=B_SPLINE_CURVE_WITH_KNOTS('',3,(#45399,#45400,#45401,#45402),
 .UNSPECIFIED.,.F.,.F.,(4,4),(1.32762608770811,1.39069260388053),
 .UNSPECIFIED.);
#1031=B_SPLINE_CURVE_WITH_KNOTS('',3,(#45403,#45404,#45405,#45406,#45407,
#45408),.UNSPECIFIED.,.F.,.F.,(4,1,1,4),(13.9260590743719,14.6127190316793,
15.6070601843597,15.7079632679489),.UNSPECIFIED.);
#1032=B_SPLINE_CURVE_WITH_KNOTS('',3,(#45924,#45925,#45926,#45927,#45928,
#45929,#45930,#45931,#45932,#45933),.UNSPECIFIED.,.F.,.F.,(4,2,2,2,4),(0.,
0.0922653926040451,0.19687474867418,0.27592539811023,0.366392236014044),
 .UNSPECIFIED.);
#1033=B_SPLINE_CURVE_WITH_KNOTS('',3,(#45934,#45935,#45936,#45937,#45938,
#45939,#45940,#45941,#45942,#45943,#45944,#45945,#45946,#45947,#45948,#45949,
#45950,#45951,#45952,#45953,#45954,#45955),.UNSPECIFIED.,.F.,.F.,(4,3,3,
3,3,3,3,4),(-10.1321597128207,-9.71411823813461,-8.71977708545417,-7.72543593277374,
-6.7310947800933,-5.73675362741286,-4.74241247473242,-3.84897440564112),
 .UNSPECIFIED.);
#1034=B_SPLINE_CURVE_WITH_KNOTS('',3,(#45956,#45957,#45958,#45959,#45960,
#45961,#45962,#45963,#45964,#45965,#45966,#45967,#45968,#45969,#45970,#45971,
#45972,#45973,#45974,#45975,#45976,#45977,#45978,#45979,#45980,#45981,#45982,
#45983,#45984,#45985,#45986,#45987,#45988,#45989,#45990,#45991,#45992,#45993,
#45994,#45995,#45996,#45997,#45998,#45999,#46000,#46001,#46002,#46003,#46004,
#46005,#46006,#46007,#46008,#46009,#46010,#46011,#46012,#46013,#46014,#46015,
#46016,#46017,#46018,#46019,#46020,#46021,#46022,#46023,#46024,#46025,#46026,
#46027,#46028,#46029,#46030,#46031,#46032,#46033,#46034,#46035,#46036,#46037,
#46038,#46039,#46040,#46041,#46042,#46043,#46044,#46045,#46046,#46047,#46048,
#46049),.UNSPECIFIED.,.F.,.F.,(4,3,3,3,3,3,3,3,3,3,3,3,3,3,3,3,3,3,3,3,
3,3,3,3,3,3,3,3,3,3,3,4),(-0.566847306048092,-0.536659932336638,-0.506051628309191,
-0.497421280406101,-0.490480107277087,-0.460332319899778,-0.437026301553265,
-0.424536425828322,-0.419839798678714,-0.39041568100221,-0.361282804033577,
-0.332973937139576,-0.318201496136602,-0.312453900617058,-0.308226501095536,
-0.280245932615023,-0.273884173127677,-0.245401703722135,-0.215623103089417,
-0.205167690233524,-0.200844138142904,-0.173009394645689,-0.1452391401898,
-0.117941713188566,-0.104095611372543,-0.0998982711600488,-0.0958071190833449,
-0.0691345029495114,-0.0429122063821633,-0.0175007642606556,-0.00717289866038673,
0.),.UNSPECIFIED.);
#1035=B_SPLINE_CURVE_WITH_KNOTS('',3,(#46050,#46051,#46052,#46053,#46054,
#46055,#46056,#46057,#46058,#46059),.UNSPECIFIED.,.F.,.F.,(4,1,1,1,1,1,
1,4),(15.7079632679489,16.6014013370402,17.5957424897206,18.590083642401,
19.5844247950815,20.5787659477619,21.5731071004423,21.9911485751284),
 .UNSPECIFIED.);
#1036=B_SPLINE_CURVE_WITH_KNOTS('',3,(#46061,#46062,#46063,#46064,#46065,
#46066,#46067,#46068,#46069,#46070),.UNSPECIFIED.,.F.,.F.,(4,1,1,1,1,1,
1,4),(15.7079632679489,16.481671388406,17.4731714687642,18.4646715491223,
19.4561716294804,20.4476717098386,21.4391717901967,21.9911485751284),
 .UNSPECIFIED.);
#1037=B_SPLINE_CURVE_WITH_KNOTS('',3,(#46543,#46544,#46545,#46546,#46547,
#46548,#46549,#46550,#46551,#46552,#46553,#46554,#46555,#46556,#46557,#46558,
#46559,#46560,#46561,#46562,#46563,#46564,#46565,#46566,#46567,#46568,#46569,
#46570,#46571,#46572,#46573,#46574,#46575,#46576,#46577,#46578,#46579,#46580,
#46581,#46582,#46583,#46584,#46585,#46586,#46587,#46588,#46589,#46590,#46591),
 .UNSPECIFIED.,.F.,.F.,(4,3,3,3,3,3,3,3,3,3,3,3,3,3,3,3,4),(0.,0.0248791739331723,
0.0501121717718979,0.0650752050475519,0.0910593995310815,0.117735388481178,
0.1391452357804,0.166055098965252,0.193202261006004,0.220029692886475,0.225091895299352,
0.25325494877503,0.279552389918125,0.281418002250707,0.290257524611623,
0.319505113634681,0.339076691562976),.UNSPECIFIED.);
#1038=B_SPLINE_CURVE_WITH_KNOTS('',3,(#46592,#46593,#46594,#46595,#46596,
#46597,#46598,#46599,#46600,#46601,#46602,#46603,#46604,#46605,#46606,#46607,
#46608,#46609,#46610,#46611,#46612,#46613,#46614,#46615,#46616,#46617,#46618,
#46619,#46620,#46621,#46622,#46623,#46624,#46625,#46626,#46627,#46628,#46629,
#46630,#46631,#46632,#46633,#46634,#46635,#46636,#46637,#46638,#46639,#46640,
#46641,#46642,#46643,#46644,#46645,#46646,#46647,#46648,#46649,#46650,#46651,
#46652,#46653,#46654,#46655,#46656,#46657,#46658,#46659,#46660,#46661,#46662,
#46663,#46664,#46665,#46666,#46667,#46668,#46669,#46670,#46671,#46672,#46673,
#46674,#46675,#46676,#46677,#46678,#46679,#46680,#46681,#46682,#46683,#46684,
#46685,#46686,#46687,#46688),.UNSPECIFIED.,.F.,.F.,(4,3,3,3,3,3,3,3,3,3,
3,3,3,3,3,3,3,3,3,3,3,3,3,3,3,3,3,3,3,3,3,3,4),(-0.569248610399451,-0.543564147881696,
-0.517253215506404,-0.5103603769831,-0.504797172077816,-0.477729530540692,
-0.455926184899551,-0.447499120623838,-0.442666727878697,-0.414934144456378,
-0.386773112743309,-0.358832030543205,-0.344949714260295,-0.340765289286146,
-0.336287711713791,-0.3073583091604,-0.303302765411564,-0.275496663855623,
-0.247058322334847,-0.237724074505435,-0.232212001847737,-0.227959645025499,
-0.198971930287922,-0.169410328510115,-0.139612457779761,-0.123469388622888,
-0.118279464491879,-0.114057511149134,-0.0835165944488132,-0.0529401030670342,
-0.0229717557625582,-0.01046790452478,0.),.UNSPECIFIED.);
#1039=B_SPLINE_CURVE_WITH_KNOTS('',3,(#46689,#46690,#46691,#46692,#46693,
#46694,#46695,#46696,#46697,#46698,#46699,#46700,#46701,#46702,#46703,#46704,
#46705,#46706,#46707,#46708,#46709,#46710),.UNSPECIFIED.,.F.,.F.,(4,3,3,
3,3,3,3,4),(7.59274844815659,8.03227174358307,9.0237718239412,10.0152719042993,
11.0067719846575,11.9982720650156,12.9897721453737,13.8759337553362),
 .UNSPECIFIED.);
#1558=SHAPE_REPRESENTATION_RELATIONSHIP('SRR','None',#63997,#1576);
#1576=ADVANCED_BREP_SHAPE_REPRESENTATION('',(#1612),#63882);
#1594=STYLED_ITEM('',(#64096),#1612);
#1612=MANIFOLD_SOLID_BREP('Body1',#15480);
#1661=FACE_BOUND('',#3976,.T.);
#1662=FACE_BOUND('',#3978,.T.);
#1663=FACE_BOUND('',#3985,.T.);
#1664=FACE_BOUND('',#3997,.T.);
#1665=FACE_BOUND('',#3999,.T.);
#1666=FACE_BOUND('',#4003,.T.);
#1667=FACE_BOUND('',#4005,.T.);
#1668=FACE_BOUND('',#4007,.T.);
#2060=CYLINDRICAL_SURFACE('',#16185,2.5175);
#2061=CYLINDRICAL_SURFACE('',#16188,2.5175);
#2062=CYLINDRICAL_SURFACE('',#16189,2.5175);
#2063=CYLINDRICAL_SURFACE('',#16190,2.5175);
#2064=CYLINDRICAL_SURFACE('',#16191,2.5175);
#2065=CYLINDRICAL_SURFACE('',#16192,2.5175);
#2066=CYLINDRICAL_SURFACE('',#16193,2.5175);
#2067=CYLINDRICAL_SURFACE('',#16194,2.5175);
#2068=CYLINDRICAL_SURFACE('',#16195,2.5175);
#2069=CYLINDRICAL_SURFACE('',#16196,2.5175);
#2070=CYLINDRICAL_SURFACE('',#16197,2.5175);
#2071=CYLINDRICAL_SURFACE('',#16198,2.5175);
#2072=CYLINDRICAL_SURFACE('',#16199,2.5175);
#2073=CYLINDRICAL_SURFACE('',#16200,2.5175);
#2074=CYLINDRICAL_SURFACE('',#16201,2.5175);
#2075=CYLINDRICAL_SURFACE('',#16202,2.5175);
#2076=CYLINDRICAL_SURFACE('',#16203,2.5175);
#2077=CYLINDRICAL_SURFACE('',#16204,2.5175);
#2078=CYLINDRICAL_SURFACE('',#16205,3.0735);
#2079=CYLINDRICAL_SURFACE('',#16208,3.0735);
#2080=CYLINDRICAL_SURFACE('',#16209,3.0735);
#2081=CYLINDRICAL_SURFACE('',#16210,3.0735);
#2082=CYLINDRICAL_SURFACE('',#16211,3.0735);
#2083=CYLINDRICAL_SURFACE('',#16212,3.0735);
#2084=CYLINDRICAL_SURFACE('',#16213,3.0735);
#2085=CYLINDRICAL_SURFACE('',#16214,3.0735);
#2086=CYLINDRICAL_SURFACE('',#16215,3.0735);
#2087=CYLINDRICAL_SURFACE('',#16216,3.0735);
#2088=CYLINDRICAL_SURFACE('',#16217,3.0735);
#2089=CYLINDRICAL_SURFACE('',#16218,3.0735);
#2090=CYLINDRICAL_SURFACE('',#16219,3.0735);
#2091=CYLINDRICAL_SURFACE('',#16220,3.0735);
#2092=CYLINDRICAL_SURFACE('',#16221,3.0735);
#2093=CYLINDRICAL_SURFACE('',#16222,3.0735);
#2094=CYLINDRICAL_SURFACE('',#16223,3.0735);
#2095=CYLINDRICAL_SURFACE('',#16224,3.0735);
#2096=CYLINDRICAL_SURFACE('',#16225,19.);
#2097=CYLINDRICAL_SURFACE('',#16232,20.);
#2098=CYLINDRICAL_SURFACE('',#16242,3.0735);
#2099=CYLINDRICAL_SURFACE('',#16244,2.5175);
#2100=CYLINDRICAL_SURFACE('',#16246,8.);
#2101=CYLINDRICAL_SURFACE('',#16250,12.);
#2102=CYLINDRICAL_SURFACE('',#16259,26.);
#2103=CYLINDRICAL_SURFACE('',#16260,20.);
#2104=CYLINDRICAL_SURFACE('',#16264,26.);
#2105=CYLINDRICAL_SURFACE('',#16267,20.);
#2477=CIRCLE('',#16186,2.5175);
#2478=CIRCLE('',#16187,2.5175);
#2479=CIRCLE('',#16206,3.0735);
#2480=CIRCLE('',#16207,3.0735);
#2481=CIRCLE('',#16226,19.);
#2482=CIRCLE('',#16227,19.);
#2483=CIRCLE('',#16229,20.);
#2484=CIRCLE('',#16231,20.);
#2485=CIRCLE('',#16233,20.);
#2486=CIRCLE('',#16237,12.);
#2487=CIRCLE('',#16240,12.);
#2488=CIRCLE('',#16241,12.);
#2489=CIRCLE('',#16247,8.);
#2490=CIRCLE('',#16248,8.);
#2491=CIRCLE('',#16251,12.);
#2492=CIRCLE('',#16254,26.);
#2493=CIRCLE('',#16255,20.);
#2494=CIRCLE('',#16257,26.);
#2495=CIRCLE('',#16258,20.);
#2496=CIRCLE('',#16261,20.);
#2497=CIRCLE('',#16263,26.);
#2498=CIRCLE('',#16265,26.);
#3067=FACE_OUTER_BOUND('',#3938,.T.);
#3068=FACE_OUTER_BOUND('',#3939,.T.);
#3069=FACE_OUTER_BOUND('',#3940,.T.);
#3070=FACE_OUTER_BOUND('',#3941,.T.);
#3071=FACE_OUTER_BOUND('',#3942,.T.);
#3072=FACE_OUTER_BOUND('',#3943,.T.);
#3073=FACE_OUTER_BOUND('',#3944,.T.);
#3074=FACE_OUTER_BOUND('',#3945,.T.);
#3075=FACE_OUTER_BOUND('',#3946,.T.);
#3076=FACE_OUTER_BOUND('',#3947,.T.);
#3077=FACE_OUTER_BOUND('',#3948,.T.);
#3078=FACE_OUTER_BOUND('',#3949,.T.);
#3079=FACE_OUTER_BOUND('',#3950,.T.);
#3080=FACE_OUTER_BOUND('',#3951,.T.);
#3081=FACE_OUTER_BOUND('',#3952,.T.);
#3082=FACE_OUTER_BOUND('',#3953,.T.);
#3083=FACE_OUTER_BOUND('',#3954,.T.);
#3084=FACE_OUTER_BOUND('',#3955,.T.);
#3085=FACE_OUTER_BOUND('',#3956,.T.);
#3086=FACE_OUTER_BOUND('',#3957,.T.);
#3087=FACE_OUTER_BOUND('',#3958,.T.);
#3088=FACE_OUTER_BOUND('',#3959,.T.);
#3089=FACE_OUTER_BOUND('',#3960,.T.);
#3090=FACE_OUTER_BOUND('',#3961,.T.);
#3091=FACE_OUTER_BOUND('',#3962,.T.);
#3092=FACE_OUTER_BOUND('',#3963,.T.);
#3093=FACE_OUTER_BOUND('',#3964,.T.);
#3094=FACE_OUTER_BOUND('',#3965,.T.);
#3095=FACE_OUTER_BOUND('',#3966,.T.);
#3096=FACE_OUTER_BOUND('',#3967,.T.);
#3097=FACE_OUTER_BOUND('',#3968,.T.);
#3098=FACE_OUTER_BOUND('',#3969,.T.);
#3099=FACE_OUTER_BOUND('',#3970,.T.);
#3100=FACE_OUTER_BOUND('',#3971,.T.);
#3101=FACE_OUTER_BOUND('',#3972,.T.);
#3102=FACE_OUTER_BOUND('',#3973,.T.);
#3103=FACE_OUTER_BOUND('',#3974,.T.);
#3104=FACE_OUTER_BOUND('',#3975,.T.);
#3105=FACE_OUTER_BOUND('',#3977,.T.);
#3106=FACE_OUTER_BOUND('',#3979,.T.);
#3107=FACE_OUTER_BOUND('',#3980,.T.);
#3108=FACE_OUTER_BOUND('',#3981,.T.);
#3109=FACE_OUTER_BOUND('',#3982,.T.);
#3110=FACE_OUTER_BOUND('',#3983,.T.);
#3111=FACE_OUTER_BOUND('',#3984,.T.);
#3112=FACE_OUTER_BOUND('',#3986,.T.);
#3113=FACE_OUTER_BOUND('',#3987,.T.);
#3114=FACE_OUTER_BOUND('',#3988,.T.);
#3115=FACE_OUTER_BOUND('',#3989,.T.);
#3116=FACE_OUTER_BOUND('',#3990,.T.);
#3117=FACE_OUTER_BOUND('',#3991,.T.);
#3118=FACE_OUTER_BOUND('',#3992,.T.);
#3119=FACE_OUTER_BOUND('',#3993,.T.);
#3120=FACE_OUTER_BOUND('',#3994,.T.);
#3121=FACE_OUTER_BOUND('',#3995,.T.);
#3122=FACE_OUTER_BOUND('',#3996,.T.);
#3123=FACE_OUTER_BOUND('',#3998,.T.);
#3124=FACE_OUTER_BOUND('',#4000,.T.);
#3125=FACE_OUTER_BOUND('',#4001,.T.);
#3126=FACE_OUTER_BOUND('',#4002,.T.);
#3127=FACE_OUTER_BOUND('',#4004,.T.);
#3128=FACE_OUTER_BOUND('',#4006,.T.);
#3129=FACE_OUTER_BOUND('',#4008,.T.);
#3938=EDGE_LOOP('',(#12172,#12173,#12174,#12175,#12176));
#3939=EDGE_LOOP('',(#12177,#12178,#12179,#12180));
#3940=EDGE_LOOP('',(#12181,#12182,#12183,#12184));
#3941=EDGE_LOOP('',(#12185,#12186,#12187,#12188));
#3942=EDGE_LOOP('',(#12189,#12190,#12191,#12192));
#3943=EDGE_LOOP('',(#12193,#12194,#12195,#12196));
#3944=EDGE_LOOP('',(#12197,#12198,#12199,#12200));
#3945=EDGE_LOOP('',(#12201,#12202,#12203,#12204));
#3946=EDGE_LOOP('',(#12205,#12206,#12207,#12208));
#3947=EDGE_LOOP('',(#12209,#12210,#12211,#12212));
#3948=EDGE_LOOP('',(#12213,#12214,#12215,#12216));
#3949=EDGE_LOOP('',(#12217,#12218,#12219,#12220));
#3950=EDGE_LOOP('',(#12221,#12222,#12223,#12224));
#3951=EDGE_LOOP('',(#12225,#12226,#12227,#12228));
#3952=EDGE_LOOP('',(#12229,#12230,#12231,#12232));
#3953=EDGE_LOOP('',(#12233,#12234,#12235,#12236));
#3954=EDGE_LOOP('',(#12237,#12238,#12239,#12240));
#3955=EDGE_LOOP('',(#12241,#12242,#12243,#12244));
#3956=EDGE_LOOP('',(#12245,#12246,#12247,#12248,#12249));
#3957=EDGE_LOOP('',(#12250,#12251,#12252,#12253));
#3958=EDGE_LOOP('',(#12254,#12255,#12256,#12257));
#3959=EDGE_LOOP('',(#12258,#12259,#12260,#12261));
#3960=EDGE_LOOP('',(#12262,#12263,#12264,#12265));
#3961=EDGE_LOOP('',(#12266,#12267,#12268,#12269));
#3962=EDGE_LOOP('',(#12270,#12271,#12272,#12273));
#3963=EDGE_LOOP('',(#12274,#12275,#12276,#12277));
#3964=EDGE_LOOP('',(#12278,#12279,#12280,#12281));
#3965=EDGE_LOOP('',(#12282,#12283,#12284,#12285));
#3966=EDGE_LOOP('',(#12286,#12287,#12288,#12289));
#3967=EDGE_LOOP('',(#12290,#12291,#12292,#12293));
#3968=EDGE_LOOP('',(#12294,#12295,#12296,#12297));
#3969=EDGE_LOOP('',(#12298,#12299,#12300,#12301));
#3970=EDGE_LOOP('',(#12302,#12303,#12304,#12305));
#3971=EDGE_LOOP('',(#12306,#12307,#12308,#12309));
#3972=EDGE_LOOP('',(#12310,#12311,#12312,#12313));
#3973=EDGE_LOOP('',(#12314,#12315,#12316,#12317,#12318));
#3974=EDGE_LOOP('',(#12319,#12320,#12321,#12322));
#3975=EDGE_LOOP('',(#12323));
#3976=EDGE_LOOP('',(#12324));
#3977=EDGE_LOOP('',(#12325));
#3978=EDGE_LOOP('',(#12326));
#3979=EDGE_LOOP('',(#12327,#12328,#12329,#12330));
#3980=EDGE_LOOP('',(#12331,#12332,#12333,#12334));
#3981=EDGE_LOOP('',(#12335,#12336,#12337,#12338));
#3982=EDGE_LOOP('',(#12339,#12340,#12341,#12342));
#3983=EDGE_LOOP('',(#12343,#12344,#12345,#12346));
#3984=EDGE_LOOP('',(#12347));
#3985=EDGE_LOOP('',(#12348,#12349,#12350,#12351,#12352));
#3986=EDGE_LOOP('',(#12353,#12354,#12355,#12356,#12357,#12358,#12359,#12360,
#12361,#12362,#12363,#12364,#12365,#12366,#12367,#12368,#12369,#12370,#12371,
#12372,#12373,#12374,#12375,#12376,#12377,#12378,#12379,#12380,#12381,#12382,
#12383,#12384,#12385,#12386,#12387,#12388,#12389,#12390,#12391,#12392));
#3987=EDGE_LOOP('',(#12393,#12394,#12395,#12396));
#3988=EDGE_LOOP('',(#12397,#12398,#12399,#12400,#12401,#12402,#12403,#12404,
#12405,#12406,#12407,#12408,#12409,#12410,#12411,#12412,#12413,#12414,#12415,
#12416,#12417,#12418,#12419,#12420,#12421,#12422,#12423,#12424,#12425,#12426,
#12427,#12428,#12429,#12430,#12431,#12432,#12433,#12434,#12435,#12436));
#3989=EDGE_LOOP('',(#12437,#12438,#12439,#12440));
#3990=EDGE_LOOP('',(#12441,#12442,#12443,#12444));
#3991=EDGE_LOOP('',(#12445,#12446,#12447,#12448));
#3992=EDGE_LOOP('',(#12449,#12450,#12451,#12452,#12453,#12454,#12455,#12456));
#3993=EDGE_LOOP('',(#12457));
#3994=EDGE_LOOP('',(#12458,#12459,#12460,#12461,#12462,#12463,#12464,#12465));
#3995=EDGE_LOOP('',(#12466));
#3996=EDGE_LOOP('',(#12467));
#3997=EDGE_LOOP('',(#12468));
#3998=EDGE_LOOP('',(#12469));
#3999=EDGE_LOOP('',(#12470));
#4000=EDGE_LOOP('',(#12471,#12472,#12473,#12474));
#4001=EDGE_LOOP('',(#12475,#12476,#12477,#12478));
#4002=EDGE_LOOP('',(#12479));
#4003=EDGE_LOOP('',(#12480));
#4004=EDGE_LOOP('',(#12481,#12482,#12483,#12484));
#4005=EDGE_LOOP('',(#12485,#12486,#12487,#12488,#12489));
#4006=EDGE_LOOP('',(#12490));
#4007=EDGE_LOOP('',(#12491));
#4008=EDGE_LOOP('',(#12492,#12493,#12494,#12495));
#4799=LINE('',#44083,#5562);
#4800=LINE('',#44106,#5563);
#4801=LINE('',#44157,#5564);
#4802=LINE('',#44208,#5565);
#4803=LINE('',#44256,#5566);
#4804=LINE('',#44307,#5567);
#4805=LINE('',#44358,#5568);
#4806=LINE('',#44406,#5569);
#4807=LINE('',#44457,#5570);
#4808=LINE('',#44508,#5571);
#4809=LINE('',#44556,#5572);
#4810=LINE('',#44607,#5573);
#4811=LINE('',#44655,#5574);
#4812=LINE('',#44706,#5575);
#4813=LINE('',#44757,#5576);
#4814=LINE('',#44805,#5577);
#4815=LINE('',#44856,#5578);
#4816=LINE('',#44907,#5579);
#4817=LINE('',#44961,#5580);
#4818=LINE('',#44987,#5581);
#4819=LINE('',#45011,#5582);
#4820=LINE('',#45036,#5583);
#4821=LINE('',#45061,#5584);
#4822=LINE('',#45085,#5585);
#4823=LINE('',#45110,#5586);
#4824=LINE('',#45135,#5587);
#4825=LINE('',#45159,#5588);
#4826=LINE('',#45184,#5589);
#4827=LINE('',#45209,#5590);
#4828=LINE('',#45233,#5591);
#4829=LINE('',#45257,#5592);
#4830=LINE('',#45283,#5593);
#4831=LINE('',#45307,#5594);
#4832=LINE('',#45331,#5595);
#4833=LINE('',#45357,#5596);
#4834=LINE('',#45381,#5597);
#4835=LINE('',#45413,#5598);
#4836=LINE('',#45424,#5599);
#4837=LINE('',#45428,#5600);
#4838=LINE('',#45430,#5601);
#4839=LINE('',#45432,#5602);
#4840=LINE('',#45433,#5603);
#4841=LINE('',#45436,#5604);
#4842=LINE('',#45438,#5605);
#4843=LINE('',#45439,#5606);
#4844=LINE('',#45443,#5607);
#4845=LINE('',#45446,#5608);
#4846=LINE('',#45447,#5609);
#4847=LINE('',#46712,#5610);
#4848=LINE('',#46715,#5611);
#4849=LINE('',#46719,#5612);
#4850=LINE('',#46721,#5613);
#4851=LINE('',#46727,#5614);
#4852=LINE('',#46740,#5615);
#4853=LINE('',#46743,#5616);
#4854=LINE('',#46750,#5617);
#4855=LINE('',#46754,#5618);
#5562=VECTOR('',#18217,3.);
#5563=VECTOR('',#18224,3.);
#5564=VECTOR('',#18227,3.);
#5565=VECTOR('',#18230,3.);
#5566=VECTOR('',#18233,3.);
#5567=VECTOR('',#18236,3.);
#5568=VECTOR('',#18239,3.);
#5569=VECTOR('',#18242,3.);
#5570=VECTOR('',#18245,3.);
#5571=VECTOR('',#18248,3.);
#5572=VECTOR('',#18251,3.);
#5573=VECTOR('',#18254,3.);
#5574=VECTOR('',#18257,3.);
#5575=VECTOR('',#18260,3.);
#5576=VECTOR('',#18263,3.);
#5577=VECTOR('',#18266,3.);
#5578=VECTOR('',#18269,3.);
#5579=VECTOR('',#18272,3.);
#5580=VECTOR('',#18275,3.0735);
#5581=VECTOR('',#18282,3.0735);
#5582=VECTOR('',#18285,3.0735);
#5583=VECTOR('',#18288,3.0735);
#5584=VECTOR('',#18291,3.0735);
#5585=VECTOR('',#18294,3.0735);
#5586=VECTOR('',#18297,3.0735);
#5587=VECTOR('',#18300,3.0735);
#5588=VECTOR('',#18303,3.0735);
#5589=VECTOR('',#18306,3.0735);
#5590=VECTOR('',#18309,3.0735);
#5591=VECTOR('',#18312,3.0735);
#5592=VECTOR('',#18315,3.0735);
#5593=VECTOR('',#18318,3.0735);
#5594=VECTOR('',#18321,3.0735);
#5595=VECTOR('',#18324,3.0735);
#5596=VECTOR('',#18327,3.0735);
#5597=VECTOR('',#18330,3.0735);
#5598=VECTOR('',#18335,19.);
#5599=VECTOR('',#18350,20.);
#5600=VECTOR('',#18353,10.);
#5601=VECTOR('',#18354,10.);
#5602=VECTOR('',#18355,10.);
#5603=VECTOR('',#18356,10.);
#5604=VECTOR('',#18359,10.);
#5605=VECTOR('',#18360,10.);
#5606=VECTOR('',#18361,10.);
#5607=VECTOR('',#18366,10.);
#5608=VECTOR('',#18369,10.);
#5609=VECTOR('',#18370,10.);
#5610=VECTOR('',#18381,10.);
#5611=VECTOR('',#18386,10.);
#5612=VECTOR('',#18391,8.);
#5613=VECTOR('',#18392,8.);
#5614=VECTOR('',#18401,12.);
#5615=VECTOR('',#18418,26.);
#5616=VECTOR('',#18421,20.);
#5617=VECTOR('',#18430,26.);
#5618=VECTOR('',#18437,20.);
#6725=VERTEX_POINT('',#44081);
#6726=VERTEX_POINT('',#44082);
#6727=VERTEX_POINT('',#44084);
#6728=VERTEX_POINT('',#44089);
#6729=VERTEX_POINT('',#44091);
#6730=VERTEX_POINT('',#44104);
#6731=VERTEX_POINT('',#44105);
#6732=VERTEX_POINT('',#44155);
#6733=VERTEX_POINT('',#44156);
#6734=VERTEX_POINT('',#44206);
#6735=VERTEX_POINT('',#44207);
#6736=VERTEX_POINT('',#44254);
#6737=VERTEX_POINT('',#44255);
#6738=VERTEX_POINT('',#44305);
#6739=VERTEX_POINT('',#44306);
#6740=VERTEX_POINT('',#44356);
#6741=VERTEX_POINT('',#44357);
#6742=VERTEX_POINT('',#44404);
#6743=VERTEX_POINT('',#44405);
#6744=VERTEX_POINT('',#44455);
#6745=VERTEX_POINT('',#44456);
#6746=VERTEX_POINT('',#44506);
#6747=VERTEX_POINT('',#44507);
#6748=VERTEX_POINT('',#44554);
#6749=VERTEX_POINT('',#44555);
#6750=VERTEX_POINT('',#44605);
#6751=VERTEX_POINT('',#44606);
#6752=VERTEX_POINT('',#44653);
#6753=VERTEX_POINT('',#44654);
#6754=VERTEX_POINT('',#44704);
#6755=VERTEX_POINT('',#44705);
#6756=VERTEX_POINT('',#44755);
#6757=VERTEX_POINT('',#44756);
#6758=VERTEX_POINT('',#44803);
#6759=VERTEX_POINT('',#44804);
#6760=VERTEX_POINT('',#44854);
#6761=VERTEX_POINT('',#44855);
#6762=VERTEX_POINT('',#44905);
#6763=VERTEX_POINT('',#44906);
#6764=VERTEX_POINT('',#44908);
#6765=VERTEX_POINT('',#44922);
#6766=VERTEX_POINT('',#44959);
#6767=VERTEX_POINT('',#44960);
#6768=VERTEX_POINT('',#44962);
#6769=VERTEX_POINT('',#44971);
#6770=VERTEX_POINT('',#44973);
#6771=VERTEX_POINT('',#44985);
#6772=VERTEX_POINT('',#44986);
#6773=VERTEX_POINT('',#45009);
#6774=VERTEX_POINT('',#45010);
#6775=VERTEX_POINT('',#45034);
#6776=VERTEX_POINT('',#45035);
#6777=VERTEX_POINT('',#45059);
#6778=VERTEX_POINT('',#45060);
#6779=VERTEX_POINT('',#45083);
#6780=VERTEX_POINT('',#45084);
#6781=VERTEX_POINT('',#45108);
#6782=VERTEX_POINT('',#45109);
#6783=VERTEX_POINT('',#45133);
#6784=VERTEX_POINT('',#45134);
#6785=VERTEX_POINT('',#45157);
#6786=VERTEX_POINT('',#45158);
#6787=VERTEX_POINT('',#45182);
#6788=VERTEX_POINT('',#45183);
#6789=VERTEX_POINT('',#45207);
#6790=VERTEX_POINT('',#45208);
#6791=VERTEX_POINT('',#45231);
#6792=VERTEX_POINT('',#45232);
#6793=VERTEX_POINT('',#45255);
#6794=VERTEX_POINT('',#45256);
#6795=VERTEX_POINT('',#45281);
#6796=VERTEX_POINT('',#45282);
#6797=VERTEX_POINT('',#45305);
#6798=VERTEX_POINT('',#45306);
#6799=VERTEX_POINT('',#45329);
#6800=VERTEX_POINT('',#45330);
#6801=VERTEX_POINT('',#45355);
#6802=VERTEX_POINT('',#45356);
#6803=VERTEX_POINT('',#45379);
#6804=VERTEX_POINT('',#45380);
#6805=VERTEX_POINT('',#45382);
#6806=VERTEX_POINT('',#45387);
#6807=VERTEX_POINT('',#45398);
#6808=VERTEX_POINT('',#45410);
#6809=VERTEX_POINT('',#45412);
#6810=VERTEX_POINT('',#45416);
#6811=VERTEX_POINT('',#45419);
#6812=VERTEX_POINT('',#45422);
#6813=VERTEX_POINT('',#45426);
#6814=VERTEX_POINT('',#45427);
#6815=VERTEX_POINT('',#45429);
#6816=VERTEX_POINT('',#45431);
#6817=VERTEX_POINT('',#45435);
#6818=VERTEX_POINT('',#45437);
#6819=VERTEX_POINT('',#45441);
#6820=VERTEX_POINT('',#45445);
#6821=VERTEX_POINT('',#45449);
#6822=VERTEX_POINT('',#46717);
#6823=VERTEX_POINT('',#46720);
#6824=VERTEX_POINT('',#46725);
#6825=VERTEX_POINT('',#46730);
#6826=VERTEX_POINT('',#46732);
#6827=VERTEX_POINT('',#46735);
#6828=VERTEX_POINT('',#46737);
#6829=VERTEX_POINT('',#46742);
#6830=VERTEX_POINT('',#46746);
#6831=VERTEX_POINT('',#46749);
#8675=EDGE_CURVE('',#6725,#6726,#4799,.T.);
#8676=EDGE_CURVE('',#6726,#6727,#957,.T.);
#8677=EDGE_CURVE('',#6727,#6728,#2477,.F.);
#8678=EDGE_CURVE('',#6728,#6729,#2478,.F.);
#8679=EDGE_CURVE('',#6729,#6725,#958,.T.);
#8680=EDGE_CURVE('',#6730,#6731,#4800,.T.);
#8681=EDGE_CURVE('',#6731,#6726,#959,.T.);
#8682=EDGE_CURVE('',#6725,#6730,#960,.T.);
#8683=EDGE_CURVE('',#6732,#6733,#4801,.T.);
#8684=EDGE_CURVE('',#6733,#6731,#961,.T.);
#8685=EDGE_CURVE('',#6730,#6732,#962,.T.);
#8686=EDGE_CURVE('',#6734,#6735,#4802,.T.);
#8687=EDGE_CURVE('',#6735,#6733,#963,.T.);
#8688=EDGE_CURVE('',#6732,#6734,#964,.T.);
#8689=EDGE_CURVE('',#6736,#6737,#4803,.T.);
#8690=EDGE_CURVE('',#6737,#6735,#965,.T.);
#8691=EDGE_CURVE('',#6734,#6736,#966,.T.);
#8692=EDGE_CURVE('',#6738,#6739,#4804,.T.);
#8693=EDGE_CURVE('',#6739,#6737,#967,.T.);
#8694=EDGE_CURVE('',#6736,#6738,#968,.T.);
#8695=EDGE_CURVE('',#6740,#6741,#4805,.T.);
#8696=EDGE_CURVE('',#6741,#6739,#969,.T.);
#8697=EDGE_CURVE('',#6738,#6740,#970,.T.);
#8698=EDGE_CURVE('',#6742,#6743,#4806,.T.);
#8699=EDGE_CURVE('',#6743,#6741,#971,.T.);
#8700=EDGE_CURVE('',#6740,#6742,#972,.T.);
#8701=EDGE_CURVE('',#6744,#6745,#4807,.T.);
#8702=EDGE_CURVE('',#6745,#6743,#973,.T.);
#8703=EDGE_CURVE('',#6742,#6744,#974,.T.);
#8704=EDGE_CURVE('',#6746,#6747,#4808,.T.);
#8705=EDGE_CURVE('',#6747,#6745,#975,.T.);
#8706=EDGE_CURVE('',#6744,#6746,#976,.T.);
#8707=EDGE_CURVE('',#6748,#6749,#4809,.T.);
#8708=EDGE_CURVE('',#6749,#6747,#977,.T.);
#8709=EDGE_CURVE('',#6746,#6748,#978,.T.);
#8710=EDGE_CURVE('',#6750,#6751,#4810,.T.);
#8711=EDGE_CURVE('',#6751,#6749,#979,.T.);
#8712=EDGE_CURVE('',#6748,#6750,#980,.T.);
#8713=EDGE_CURVE('',#6752,#6753,#4811,.T.);
#8714=EDGE_CURVE('',#6753,#6751,#981,.T.);
#8715=EDGE_CURVE('',#6750,#6752,#982,.T.);
#8716=EDGE_CURVE('',#6754,#6755,#4812,.T.);
#8717=EDGE_CURVE('',#6755,#6753,#983,.T.);
#8718=EDGE_CURVE('',#6752,#6754,#984,.T.);
#8719=EDGE_CURVE('',#6756,#6757,#4813,.T.);
#8720=EDGE_CURVE('',#6757,#6755,#985,.T.);
#8721=EDGE_CURVE('',#6754,#6756,#986,.T.);
#8722=EDGE_CURVE('',#6758,#6759,#4814,.T.);
#8723=EDGE_CURVE('',#6759,#6757,#987,.T.);
#8724=EDGE_CURVE('',#6756,#6758,#988,.T.);
#8725=EDGE_CURVE('',#6760,#6761,#4815,.T.);
#8726=EDGE_CURVE('',#6761,#6759,#989,.T.);
#8727=EDGE_CURVE('',#6758,#6760,#990,.T.);
#8728=EDGE_CURVE('',#6762,#6763,#4816,.T.);
#8729=EDGE_CURVE('',#6762,#6764,#991,.T.);
#8730=EDGE_CURVE('',#6765,#6764,#992,.T.);
#8731=EDGE_CURVE('',#6765,#6763,#993,.T.);
#8732=EDGE_CURVE('',#6766,#6767,#4817,.T.);
#8733=EDGE_CURVE('',#6767,#6768,#994,.T.);
#8734=EDGE_CURVE('',#6769,#6768,#2479,.T.);
#8735=EDGE_CURVE('',#6770,#6769,#2480,.T.);
#8736=EDGE_CURVE('',#6766,#6770,#995,.T.);
#8737=EDGE_CURVE('',#6771,#6772,#4818,.T.);
#8738=EDGE_CURVE('',#6772,#6767,#996,.T.);
#8739=EDGE_CURVE('',#6771,#6766,#997,.T.);
#8740=EDGE_CURVE('',#6773,#6774,#4819,.T.);
#8741=EDGE_CURVE('',#6774,#6772,#998,.T.);
#8742=EDGE_CURVE('',#6773,#6771,#999,.T.);
#8743=EDGE_CURVE('',#6775,#6776,#4820,.T.);
#8744=EDGE_CURVE('',#6776,#6774,#1000,.T.);
#8745=EDGE_CURVE('',#6775,#6773,#1001,.T.);
#8746=EDGE_CURVE('',#6777,#6778,#4821,.T.);
#8747=EDGE_CURVE('',#6778,#6776,#1002,.T.);
#8748=EDGE_CURVE('',#6777,#6775,#1003,.T.);
#8749=EDGE_CURVE('',#6779,#6780,#4822,.T.);
#8750=EDGE_CURVE('',#6780,#6778,#1004,.T.);
#8751=EDGE_CURVE('',#6779,#6777,#1005,.T.);
#8752=EDGE_CURVE('',#6781,#6782,#4823,.T.);
#8753=EDGE_CURVE('',#6782,#6780,#1006,.T.);
#8754=EDGE_CURVE('',#6781,#6779,#1007,.T.);
#8755=EDGE_CURVE('',#6783,#6784,#4824,.T.);
#8756=EDGE_CURVE('',#6784,#6782,#1008,.T.);
#8757=EDGE_CURVE('',#6783,#6781,#1009,.T.);
#8758=EDGE_CURVE('',#6785,#6786,#4825,.T.);
#8759=EDGE_CURVE('',#6786,#6784,#1010,.T.);
#8760=EDGE_CURVE('',#6785,#6783,#1011,.T.);
#8761=EDGE_CURVE('',#6787,#6788,#4826,.T.);
#8762=EDGE_CURVE('',#6788,#6786,#1012,.T.);
#8763=EDGE_CURVE('',#6787,#6785,#1013,.T.);
#8764=EDGE_CURVE('',#6789,#6790,#4827,.T.);
#8765=EDGE_CURVE('',#6790,#6788,#1014,.T.);
#8766=EDGE_CURVE('',#6789,#6787,#1015,.T.);
#8767=EDGE_CURVE('',#6791,#6792,#4828,.T.);
#8768=EDGE_CURVE('',#6792,#6790,#1016,.T.);
#8769=EDGE_CURVE('',#6791,#6789,#1017,.T.);
#8770=EDGE_CURVE('',#6793,#6794,#4829,.T.);
#8771=EDGE_CURVE('',#6794,#6792,#1018,.T.);
#8772=EDGE_CURVE('',#6793,#6791,#1019,.T.);
#8773=EDGE_CURVE('',#6795,#6796,#4830,.T.);
#8774=EDGE_CURVE('',#6796,#6794,#1020,.T.);
#8775=EDGE_CURVE('',#6795,#6793,#1021,.T.);
#8776=EDGE_CURVE('',#6797,#6798,#4831,.T.);
#8777=EDGE_CURVE('',#6798,#6796,#1022,.T.);
#8778=EDGE_CURVE('',#6797,#6795,#1023,.T.);
#8779=EDGE_CURVE('',#6799,#6800,#4832,.T.);
#8780=EDGE_CURVE('',#6800,#6798,#1024,.T.);
#8781=EDGE_CURVE('',#6799,#6797,#1025,.T.);
#8782=EDGE_CURVE('',#6801,#6802,#4833,.T.);
#8783=EDGE_CURVE('',#6802,#6800,#1026,.T.);
#8784=EDGE_CURVE('',#6801,#6799,#1027,.T.);
#8785=EDGE_CURVE('',#6803,#6804,#4834,.T.);
#8786=EDGE_CURVE('',#6805,#6803,#1028,.T.);
#8787=EDGE_CURVE('',#6806,#6805,#1029,.T.);
#8788=EDGE_CURVE('',#6807,#6806,#1030,.T.);
#8789=EDGE_CURVE('',#6807,#6804,#1031,.T.);
#8790=EDGE_CURVE('',#6808,#6808,#2481,.T.);
#8791=EDGE_CURVE('',#6808,#6809,#4835,.T.);
#8792=EDGE_CURVE('',#6809,#6809,#2482,.T.);
#8793=EDGE_CURVE('',#6810,#6810,#2483,.T.);
#8794=EDGE_CURVE('',#6811,#6811,#2484,.T.);
#8795=EDGE_CURVE('',#6812,#6812,#2485,.T.);
#8796=EDGE_CURVE('',#6812,#6811,#4836,.T.);
#8797=EDGE_CURVE('',#6813,#6814,#4837,.T.);
#8798=EDGE_CURVE('',#6815,#6813,#4838,.T.);
#8799=EDGE_CURVE('',#6816,#6815,#4839,.T.);
#8800=EDGE_CURVE('',#6814,#6816,#4840,.T.);
#8801=EDGE_CURVE('',#6817,#6816,#4841,.T.);
#8802=EDGE_CURVE('',#6815,#6818,#4842,.T.);
#8803=EDGE_CURVE('',#6818,#6817,#4843,.T.);
#8804=EDGE_CURVE('',#6814,#6819,#2486,.T.);
#8805=EDGE_CURVE('',#6817,#6819,#4844,.T.);
#8806=EDGE_CURVE('',#6819,#6820,#4845,.T.);
#8807=EDGE_CURVE('',#6820,#6818,#4846,.T.);
#8808=EDGE_CURVE('',#6813,#6821,#2487,.T.);
#8809=EDGE_CURVE('',#6821,#6820,#2488,.T.);
#8810=EDGE_CURVE('',#6764,#6807,#1032,.T.);
#8811=EDGE_CURVE('',#6760,#6762,#1033,.T.);
#8812=EDGE_CURVE('',#6768,#6729,#1034,.T.);
#8813=EDGE_CURVE('',#6804,#6802,#1035,.T.);
#8814=EDGE_CURVE('',#6803,#6801,#1036,.T.);
#8815=EDGE_CURVE('',#6805,#6765,#1037,.T.);
#8816=EDGE_CURVE('',#6727,#6770,#1038,.T.);
#8817=EDGE_CURVE('',#6763,#6761,#1039,.T.);
#8818=EDGE_CURVE('',#6728,#6769,#4847,.T.);
#8819=EDGE_CURVE('',#6728,#6769,#4848,.T.);
#8820=EDGE_CURVE('',#6822,#6822,#2489,.T.);
#8821=EDGE_CURVE('',#6822,#6769,#4849,.T.);
#8822=EDGE_CURVE('',#6728,#6823,#4850,.T.);
#8823=EDGE_CURVE('',#6823,#6823,#2490,.T.);
#8824=EDGE_CURVE('',#6824,#6824,#2491,.T.);
#8825=EDGE_CURVE('',#6824,#6821,#4851,.T.);
#8826=EDGE_CURVE('',#6825,#6825,#2492,.T.);
#8827=EDGE_CURVE('',#6826,#6826,#2493,.T.);
#8828=EDGE_CURVE('',#6827,#6827,#2494,.T.);
#8829=EDGE_CURVE('',#6828,#6828,#2495,.T.);
#8830=EDGE_CURVE('',#6825,#6827,#4852,.T.);
#8831=EDGE_CURVE('',#6828,#6829,#4853,.T.);
#8832=EDGE_CURVE('',#6829,#6829,#2496,.T.);
#8833=EDGE_CURVE('',#6830,#6830,#2497,.T.);
#8834=EDGE_CURVE('',#6830,#6831,#4854,.T.);
#8835=EDGE_CURVE('',#6831,#6831,#2498,.T.);
#8836=EDGE_CURVE('',#6810,#6826,#4855,.T.);
#12172=ORIENTED_EDGE('',*,*,#8675,.T.);
#12173=ORIENTED_EDGE('',*,*,#8676,.T.);
#12174=ORIENTED_EDGE('',*,*,#8677,.T.);
#12175=ORIENTED_EDGE('',*,*,#8678,.T.);
#12176=ORIENTED_EDGE('',*,*,#8679,.T.);
#12177=ORIENTED_EDGE('',*,*,#8680,.T.);
#12178=ORIENTED_EDGE('',*,*,#8681,.T.);
#12179=ORIENTED_EDGE('',*,*,#8675,.F.);
#12180=ORIENTED_EDGE('',*,*,#8682,.T.);
#12181=ORIENTED_EDGE('',*,*,#8683,.T.);
#12182=ORIENTED_EDGE('',*,*,#8684,.T.);
#12183=ORIENTED_EDGE('',*,*,#8680,.F.);
#12184=ORIENTED_EDGE('',*,*,#8685,.T.);
#12185=ORIENTED_EDGE('',*,*,#8686,.T.);
#12186=ORIENTED_EDGE('',*,*,#8687,.T.);
#12187=ORIENTED_EDGE('',*,*,#8683,.F.);
#12188=ORIENTED_EDGE('',*,*,#8688,.T.);
#12189=ORIENTED_EDGE('',*,*,#8689,.T.);
#12190=ORIENTED_EDGE('',*,*,#8690,.T.);
#12191=ORIENTED_EDGE('',*,*,#8686,.F.);
#12192=ORIENTED_EDGE('',*,*,#8691,.T.);
#12193=ORIENTED_EDGE('',*,*,#8692,.T.);
#12194=ORIENTED_EDGE('',*,*,#8693,.T.);
#12195=ORIENTED_EDGE('',*,*,#8689,.F.);
#12196=ORIENTED_EDGE('',*,*,#8694,.T.);
#12197=ORIENTED_EDGE('',*,*,#8695,.T.);
#12198=ORIENTED_EDGE('',*,*,#8696,.T.);
#12199=ORIENTED_EDGE('',*,*,#8692,.F.);
#12200=ORIENTED_EDGE('',*,*,#8697,.T.);
#12201=ORIENTED_EDGE('',*,*,#8698,.T.);
#12202=ORIENTED_EDGE('',*,*,#8699,.T.);
#12203=ORIENTED_EDGE('',*,*,#8695,.F.);
#12204=ORIENTED_EDGE('',*,*,#8700,.T.);
#12205=ORIENTED_EDGE('',*,*,#8701,.T.);
#12206=ORIENTED_EDGE('',*,*,#8702,.T.);
#12207=ORIENTED_EDGE('',*,*,#8698,.F.);
#12208=ORIENTED_EDGE('',*,*,#8703,.T.);
#12209=ORIENTED_EDGE('',*,*,#8704,.T.);
#12210=ORIENTED_EDGE('',*,*,#8705,.T.);
#12211=ORIENTED_EDGE('',*,*,#8701,.F.);
#12212=ORIENTED_EDGE('',*,*,#8706,.T.);
#12213=ORIENTED_EDGE('',*,*,#8707,.T.);
#12214=ORIENTED_EDGE('',*,*,#8708,.T.);
#12215=ORIENTED_EDGE('',*,*,#8704,.F.);
#12216=ORIENTED_EDGE('',*,*,#8709,.T.);
#12217=ORIENTED_EDGE('',*,*,#8710,.T.);
#12218=ORIENTED_EDGE('',*,*,#8711,.T.);
#12219=ORIENTED_EDGE('',*,*,#8707,.F.);
#12220=ORIENTED_EDGE('',*,*,#8712,.T.);
#12221=ORIENTED_EDGE('',*,*,#8713,.T.);
#12222=ORIENTED_EDGE('',*,*,#8714,.T.);
#12223=ORIENTED_EDGE('',*,*,#8710,.F.);
#12224=ORIENTED_EDGE('',*,*,#8715,.T.);
#12225=ORIENTED_EDGE('',*,*,#8716,.T.);
#12226=ORIENTED_EDGE('',*,*,#8717,.T.);
#12227=ORIENTED_EDGE('',*,*,#8713,.F.);
#12228=ORIENTED_EDGE('',*,*,#8718,.T.);
#12229=ORIENTED_EDGE('',*,*,#8719,.T.);
#12230=ORIENTED_EDGE('',*,*,#8720,.T.);
#12231=ORIENTED_EDGE('',*,*,#8716,.F.);
#12232=ORIENTED_EDGE('',*,*,#8721,.T.);
#12233=ORIENTED_EDGE('',*,*,#8722,.T.);
#12234=ORIENTED_EDGE('',*,*,#8723,.T.);
#12235=ORIENTED_EDGE('',*,*,#8719,.F.);
#12236=ORIENTED_EDGE('',*,*,#8724,.T.);
#12237=ORIENTED_EDGE('',*,*,#8725,.T.);
#12238=ORIENTED_EDGE('',*,*,#8726,.T.);
#12239=ORIENTED_EDGE('',*,*,#8722,.F.);
#12240=ORIENTED_EDGE('',*,*,#8727,.T.);
#12241=ORIENTED_EDGE('',*,*,#8728,.F.);
#12242=ORIENTED_EDGE('',*,*,#8729,.T.);
#12243=ORIENTED_EDGE('',*,*,#8730,.F.);
#12244=ORIENTED_EDGE('',*,*,#8731,.T.);
#12245=ORIENTED_EDGE('',*,*,#8732,.T.);
#12246=ORIENTED_EDGE('',*,*,#8733,.T.);
#12247=ORIENTED_EDGE('',*,*,#8734,.F.);
#12248=ORIENTED_EDGE('',*,*,#8735,.F.);
#12249=ORIENTED_EDGE('',*,*,#8736,.F.);
#12250=ORIENTED_EDGE('',*,*,#8737,.T.);
#12251=ORIENTED_EDGE('',*,*,#8738,.T.);
#12252=ORIENTED_EDGE('',*,*,#8732,.F.);
#12253=ORIENTED_EDGE('',*,*,#8739,.F.);
#12254=ORIENTED_EDGE('',*,*,#8740,.T.);
#12255=ORIENTED_EDGE('',*,*,#8741,.T.);
#12256=ORIENTED_EDGE('',*,*,#8737,.F.);
#12257=ORIENTED_EDGE('',*,*,#8742,.F.);
#12258=ORIENTED_EDGE('',*,*,#8743,.T.);
#12259=ORIENTED_EDGE('',*,*,#8744,.T.);
#12260=ORIENTED_EDGE('',*,*,#8740,.F.);
#12261=ORIENTED_EDGE('',*,*,#8745,.F.);
#12262=ORIENTED_EDGE('',*,*,#8746,.T.);
#12263=ORIENTED_EDGE('',*,*,#8747,.T.);
#12264=ORIENTED_EDGE('',*,*,#8743,.F.);
#12265=ORIENTED_EDGE('',*,*,#8748,.F.);
#12266=ORIENTED_EDGE('',*,*,#8749,.T.);
#12267=ORIENTED_EDGE('',*,*,#8750,.T.);
#12268=ORIENTED_EDGE('',*,*,#8746,.F.);
#12269=ORIENTED_EDGE('',*,*,#8751,.F.);
#12270=ORIENTED_EDGE('',*,*,#8752,.T.);
#12271=ORIENTED_EDGE('',*,*,#8753,.T.);
#12272=ORIENTED_EDGE('',*,*,#8749,.F.);
#12273=ORIENTED_EDGE('',*,*,#8754,.F.);
#12274=ORIENTED_EDGE('',*,*,#8755,.T.);
#12275=ORIENTED_EDGE('',*,*,#8756,.T.);
#12276=ORIENTED_EDGE('',*,*,#8752,.F.);
#12277=ORIENTED_EDGE('',*,*,#8757,.F.);
#12278=ORIENTED_EDGE('',*,*,#8758,.T.);
#12279=ORIENTED_EDGE('',*,*,#8759,.T.);
#12280=ORIENTED_EDGE('',*,*,#8755,.F.);
#12281=ORIENTED_EDGE('',*,*,#8760,.F.);
#12282=ORIENTED_EDGE('',*,*,#8761,.T.);
#12283=ORIENTED_EDGE('',*,*,#8762,.T.);
#12284=ORIENTED_EDGE('',*,*,#8758,.F.);
#12285=ORIENTED_EDGE('',*,*,#8763,.F.);
#12286=ORIENTED_EDGE('',*,*,#8764,.T.);
#12287=ORIENTED_EDGE('',*,*,#8765,.T.);
#12288=ORIENTED_EDGE('',*,*,#8761,.F.);
#12289=ORIENTED_EDGE('',*,*,#8766,.F.);
#12290=ORIENTED_EDGE('',*,*,#8767,.T.);
#12291=ORIENTED_EDGE('',*,*,#8768,.T.);
#12292=ORIENTED_EDGE('',*,*,#8764,.F.);
#12293=ORIENTED_EDGE('',*,*,#8769,.F.);
#12294=ORIENTED_EDGE('',*,*,#8770,.T.);
#12295=ORIENTED_EDGE('',*,*,#8771,.T.);
#12296=ORIENTED_EDGE('',*,*,#8767,.F.);
#12297=ORIENTED_EDGE('',*,*,#8772,.F.);
#12298=ORIENTED_EDGE('',*,*,#8773,.T.);
#12299=ORIENTED_EDGE('',*,*,#8774,.T.);
#12300=ORIENTED_EDGE('',*,*,#8770,.F.);
#12301=ORIENTED_EDGE('',*,*,#8775,.F.);
#12302=ORIENTED_EDGE('',*,*,#8776,.T.);
#12303=ORIENTED_EDGE('',*,*,#8777,.T.);
#12304=ORIENTED_EDGE('',*,*,#8773,.F.);
#12305=ORIENTED_EDGE('',*,*,#8778,.F.);
#12306=ORIENTED_EDGE('',*,*,#8779,.T.);
#12307=ORIENTED_EDGE('',*,*,#8780,.T.);
#12308=ORIENTED_EDGE('',*,*,#8776,.F.);
#12309=ORIENTED_EDGE('',*,*,#8781,.F.);
#12310=ORIENTED_EDGE('',*,*,#8782,.T.);
#12311=ORIENTED_EDGE('',*,*,#8783,.T.);
#12312=ORIENTED_EDGE('',*,*,#8779,.F.);
#12313=ORIENTED_EDGE('',*,*,#8784,.F.);
#12314=ORIENTED_EDGE('',*,*,#8785,.F.);
#12315=ORIENTED_EDGE('',*,*,#8786,.F.);
#12316=ORIENTED_EDGE('',*,*,#8787,.F.);
#12317=ORIENTED_EDGE('',*,*,#8788,.F.);
#12318=ORIENTED_EDGE('',*,*,#8789,.T.);
#12319=ORIENTED_EDGE('',*,*,#8790,.T.);
#12320=ORIENTED_EDGE('',*,*,#8791,.T.);
#12321=ORIENTED_EDGE('',*,*,#8792,.F.);
#12322=ORIENTED_EDGE('',*,*,#8791,.F.);
#12323=ORIENTED_EDGE('',*,*,#8793,.F.);
#12324=ORIENTED_EDGE('',*,*,#8790,.F.);
#12325=ORIENTED_EDGE('',*,*,#8794,.F.);
#12326=ORIENTED_EDGE('',*,*,#8792,.T.);
#12327=ORIENTED_EDGE('',*,*,#8795,.F.);
#12328=ORIENTED_EDGE('',*,*,#8796,.T.);
#12329=ORIENTED_EDGE('',*,*,#8794,.T.);
#12330=ORIENTED_EDGE('',*,*,#8796,.F.);
#12331=ORIENTED_EDGE('',*,*,#8797,.F.);
#12332=ORIENTED_EDGE('',*,*,#8798,.F.);
#12333=ORIENTED_EDGE('',*,*,#8799,.F.);
#12334=ORIENTED_EDGE('',*,*,#8800,.F.);
#12335=ORIENTED_EDGE('',*,*,#8801,.T.);
#12336=ORIENTED_EDGE('',*,*,#8799,.T.);
#12337=ORIENTED_EDGE('',*,*,#8802,.T.);
#12338=ORIENTED_EDGE('',*,*,#8803,.T.);
#12339=ORIENTED_EDGE('',*,*,#8804,.F.);
#12340=ORIENTED_EDGE('',*,*,#8800,.T.);
#12341=ORIENTED_EDGE('',*,*,#8801,.F.);
#12342=ORIENTED_EDGE('',*,*,#8805,.T.);
#12343=ORIENTED_EDGE('',*,*,#8806,.F.);
#12344=ORIENTED_EDGE('',*,*,#8805,.F.);
#12345=ORIENTED_EDGE('',*,*,#8803,.F.);
#12346=ORIENTED_EDGE('',*,*,#8807,.F.);
#12347=ORIENTED_EDGE('',*,*,#8795,.T.);
#12348=ORIENTED_EDGE('',*,*,#8808,.T.);
#12349=ORIENTED_EDGE('',*,*,#8809,.T.);
#12350=ORIENTED_EDGE('',*,*,#8807,.T.);
#12351=ORIENTED_EDGE('',*,*,#8802,.F.);
#12352=ORIENTED_EDGE('',*,*,#8798,.T.);
#12353=ORIENTED_EDGE('',*,*,#8810,.F.);
#12354=ORIENTED_EDGE('',*,*,#8729,.F.);
#12355=ORIENTED_EDGE('',*,*,#8811,.F.);
#12356=ORIENTED_EDGE('',*,*,#8727,.F.);
#12357=ORIENTED_EDGE('',*,*,#8724,.F.);
#12358=ORIENTED_EDGE('',*,*,#8721,.F.);
#12359=ORIENTED_EDGE('',*,*,#8718,.F.);
#12360=ORIENTED_EDGE('',*,*,#8715,.F.);
#12361=ORIENTED_EDGE('',*,*,#8712,.F.);
#12362=ORIENTED_EDGE('',*,*,#8709,.F.);
#12363=ORIENTED_EDGE('',*,*,#8706,.F.);
#12364=ORIENTED_EDGE('',*,*,#8703,.F.);
#12365=ORIENTED_EDGE('',*,*,#8700,.F.);
#12366=ORIENTED_EDGE('',*,*,#8697,.F.);
#12367=ORIENTED_EDGE('',*,*,#8694,.F.);
#12368=ORIENTED_EDGE('',*,*,#8691,.F.);
#12369=ORIENTED_EDGE('',*,*,#8688,.F.);
#12370=ORIENTED_EDGE('',*,*,#8685,.F.);
#12371=ORIENTED_EDGE('',*,*,#8682,.F.);
#12372=ORIENTED_EDGE('',*,*,#8679,.F.);
#12373=ORIENTED_EDGE('',*,*,#8812,.F.);
#12374=ORIENTED_EDGE('',*,*,#8733,.F.);
#12375=ORIENTED_EDGE('',*,*,#8738,.F.);
#12376=ORIENTED_EDGE('',*,*,#8741,.F.);
#12377=ORIENTED_EDGE('',*,*,#8744,.F.);
#12378=ORIENTED_EDGE('',*,*,#8747,.F.);
#12379=ORIENTED_EDGE('',*,*,#8750,.F.);
#12380=ORIENTED_EDGE('',*,*,#8753,.F.);
#12381=ORIENTED_EDGE('',*,*,#8756,.F.);
#12382=ORIENTED_EDGE('',*,*,#8759,.F.);
#12383=ORIENTED_EDGE('',*,*,#8762,.F.);
#12384=ORIENTED_EDGE('',*,*,#8765,.F.);
#12385=ORIENTED_EDGE('',*,*,#8768,.F.);
#12386=ORIENTED_EDGE('',*,*,#8771,.F.);
#12387=ORIENTED_EDGE('',*,*,#8774,.F.);
#12388=ORIENTED_EDGE('',*,*,#8777,.F.);
#12389=ORIENTED_EDGE('',*,*,#8780,.F.);
#12390=ORIENTED_EDGE('',*,*,#8783,.F.);
#12391=ORIENTED_EDGE('',*,*,#8813,.F.);
#12392=ORIENTED_EDGE('',*,*,#8789,.F.);
#12393=ORIENTED_EDGE('',*,*,#8785,.T.);
#12394=ORIENTED_EDGE('',*,*,#8813,.T.);
#12395=ORIENTED_EDGE('',*,*,#8782,.F.);
#12396=ORIENTED_EDGE('',*,*,#8814,.F.);
#12397=ORIENTED_EDGE('',*,*,#8815,.F.);
#12398=ORIENTED_EDGE('',*,*,#8786,.T.);
#12399=ORIENTED_EDGE('',*,*,#8814,.T.);
#12400=ORIENTED_EDGE('',*,*,#8784,.T.);
#12401=ORIENTED_EDGE('',*,*,#8781,.T.);
#12402=ORIENTED_EDGE('',*,*,#8778,.T.);
#12403=ORIENTED_EDGE('',*,*,#8775,.T.);
#12404=ORIENTED_EDGE('',*,*,#8772,.T.);
#12405=ORIENTED_EDGE('',*,*,#8769,.T.);
#12406=ORIENTED_EDGE('',*,*,#8766,.T.);
#12407=ORIENTED_EDGE('',*,*,#8763,.T.);
#12408=ORIENTED_EDGE('',*,*,#8760,.T.);
#12409=ORIENTED_EDGE('',*,*,#8757,.T.);
#12410=ORIENTED_EDGE('',*,*,#8754,.T.);
#12411=ORIENTED_EDGE('',*,*,#8751,.T.);
#12412=ORIENTED_EDGE('',*,*,#8748,.T.);
#12413=ORIENTED_EDGE('',*,*,#8745,.T.);
#12414=ORIENTED_EDGE('',*,*,#8742,.T.);
#12415=ORIENTED_EDGE('',*,*,#8739,.T.);
#12416=ORIENTED_EDGE('',*,*,#8736,.T.);
#12417=ORIENTED_EDGE('',*,*,#8816,.F.);
#12418=ORIENTED_EDGE('',*,*,#8676,.F.);
#12419=ORIENTED_EDGE('',*,*,#8681,.F.);
#12420=ORIENTED_EDGE('',*,*,#8684,.F.);
#12421=ORIENTED_EDGE('',*,*,#8687,.F.);
#12422=ORIENTED_EDGE('',*,*,#8690,.F.);
#12423=ORIENTED_EDGE('',*,*,#8693,.F.);
#12424=ORIENTED_EDGE('',*,*,#8696,.F.);
#12425=ORIENTED_EDGE('',*,*,#8699,.F.);
#12426=ORIENTED_EDGE('',*,*,#8702,.F.);
#12427=ORIENTED_EDGE('',*,*,#8705,.F.);
#12428=ORIENTED_EDGE('',*,*,#8708,.F.);
#12429=ORIENTED_EDGE('',*,*,#8711,.F.);
#12430=ORIENTED_EDGE('',*,*,#8714,.F.);
#12431=ORIENTED_EDGE('',*,*,#8717,.F.);
#12432=ORIENTED_EDGE('',*,*,#8720,.F.);
#12433=ORIENTED_EDGE('',*,*,#8723,.F.);
#12434=ORIENTED_EDGE('',*,*,#8726,.F.);
#12435=ORIENTED_EDGE('',*,*,#8817,.F.);
#12436=ORIENTED_EDGE('',*,*,#8731,.F.);
#12437=ORIENTED_EDGE('',*,*,#8818,.T.);
#12438=ORIENTED_EDGE('',*,*,#8734,.T.);
#12439=ORIENTED_EDGE('',*,*,#8812,.T.);
#12440=ORIENTED_EDGE('',*,*,#8678,.F.);
#12441=ORIENTED_EDGE('',*,*,#8728,.T.);
#12442=ORIENTED_EDGE('',*,*,#8817,.T.);
#12443=ORIENTED_EDGE('',*,*,#8725,.F.);
#12444=ORIENTED_EDGE('',*,*,#8811,.T.);
#12445=ORIENTED_EDGE('',*,*,#8819,.F.);
#12446=ORIENTED_EDGE('',*,*,#8677,.F.);
#12447=ORIENTED_EDGE('',*,*,#8816,.T.);
#12448=ORIENTED_EDGE('',*,*,#8735,.T.);
#12449=ORIENTED_EDGE('',*,*,#8820,.F.);
#12450=ORIENTED_EDGE('',*,*,#8821,.T.);
#12451=ORIENTED_EDGE('',*,*,#8818,.F.);
#12452=ORIENTED_EDGE('',*,*,#8822,.T.);
#12453=ORIENTED_EDGE('',*,*,#8823,.T.);
#12454=ORIENTED_EDGE('',*,*,#8822,.F.);
#12455=ORIENTED_EDGE('',*,*,#8819,.T.);
#12456=ORIENTED_EDGE('',*,*,#8821,.F.);
#12457=ORIENTED_EDGE('',*,*,#8823,.F.);
#12458=ORIENTED_EDGE('',*,*,#8824,.F.);
#12459=ORIENTED_EDGE('',*,*,#8825,.T.);
#12460=ORIENTED_EDGE('',*,*,#8808,.F.);
#12461=ORIENTED_EDGE('',*,*,#8797,.T.);
#12462=ORIENTED_EDGE('',*,*,#8804,.T.);
#12463=ORIENTED_EDGE('',*,*,#8806,.T.);
#12464=ORIENTED_EDGE('',*,*,#8809,.F.);
#12465=ORIENTED_EDGE('',*,*,#8825,.F.);
#12466=ORIENTED_EDGE('',*,*,#8824,.T.);
#12467=ORIENTED_EDGE('',*,*,#8826,.T.);
#12468=ORIENTED_EDGE('',*,*,#8827,.F.);
#12469=ORIENTED_EDGE('',*,*,#8828,.F.);
#12470=ORIENTED_EDGE('',*,*,#8829,.F.);
#12471=ORIENTED_EDGE('',*,*,#8826,.F.);
#12472=ORIENTED_EDGE('',*,*,#8830,.T.);
#12473=ORIENTED_EDGE('',*,*,#8828,.T.);
#12474=ORIENTED_EDGE('',*,*,#8830,.F.);
#12475=ORIENTED_EDGE('',*,*,#8829,.T.);
#12476=ORIENTED_EDGE('',*,*,#8831,.T.);
#12477=ORIENTED_EDGE('',*,*,#8832,.T.);
#12478=ORIENTED_EDGE('',*,*,#8831,.F.);
#12479=ORIENTED_EDGE('',*,*,#8833,.T.);
#12480=ORIENTED_EDGE('',*,*,#8832,.F.);
#12481=ORIENTED_EDGE('',*,*,#8833,.F.);
#12482=ORIENTED_EDGE('',*,*,#8834,.T.);
#12483=ORIENTED_EDGE('',*,*,#8835,.T.);
#12484=ORIENTED_EDGE('',*,*,#8834,.F.);
#12485=ORIENTED_EDGE('',*,*,#8815,.T.);
#12486=ORIENTED_EDGE('',*,*,#8730,.T.);
#12487=ORIENTED_EDGE('',*,*,#8810,.T.);
#12488=ORIENTED_EDGE('',*,*,#8788,.T.);
#12489=ORIENTED_EDGE('',*,*,#8787,.T.);
#12490=ORIENTED_EDGE('',*,*,#8835,.F.);
#12491=ORIENTED_EDGE('',*,*,#8820,.T.);
#12492=ORIENTED_EDGE('',*,*,#8793,.T.);
#12493=ORIENTED_EDGE('',*,*,#8836,.T.);
#12494=ORIENTED_EDGE('',*,*,#8827,.T.);
#12495=ORIENTED_EDGE('',*,*,#8836,.F.);
#14554=PLANE('',#16228);
#14555=PLANE('',#16230);
#14556=PLANE('',#16234);
#14557=PLANE('',#16235);
#14558=PLANE('',#16236);
#14559=PLANE('',#16238);
#14560=PLANE('',#16239);
#14561=PLANE('',#16243);
#14562=PLANE('',#16245);
#14563=PLANE('',#16249);
#14564=PLANE('',#16252);
#14565=PLANE('',#16253);
#14566=PLANE('',#16256);
#14567=PLANE('',#16262);
#14568=PLANE('',#16266);
#15047=ADVANCED_FACE('',(#3067),#2060,.F.);
#15048=ADVANCED_FACE('',(#3068),#2061,.F.);
#15049=ADVANCED_FACE('',(#3069),#2062,.F.);
#15050=ADVANCED_FACE('',(#3070),#2063,.F.);
#15051=ADVANCED_FACE('',(#3071),#2064,.F.);
#15052=ADVANCED_FACE('',(#3072),#2065,.F.);
#15053=ADVANCED_FACE('',(#3073),#2066,.F.);
#15054=ADVANCED_FACE('',(#3074),#2067,.F.);
#15055=ADVANCED_FACE('',(#3075),#2068,.F.);
#15056=ADVANCED_FACE('',(#3076),#2069,.F.);
#15057=ADVANCED_FACE('',(#3077),#2070,.F.);
#15058=ADVANCED_FACE('',(#3078),#2071,.F.);
#15059=ADVANCED_FACE('',(#3079),#2072,.F.);
#15060=ADVANCED_FACE('',(#3080),#2073,.F.);
#15061=ADVANCED_FACE('',(#3081),#2074,.F.);
#15062=ADVANCED_FACE('',(#3082),#2075,.F.);
#15063=ADVANCED_FACE('',(#3083),#2076,.F.);
#15064=ADVANCED_FACE('',(#3084),#2077,.F.);
#15065=ADVANCED_FACE('',(#3085),#2078,.F.);
#15066=ADVANCED_FACE('',(#3086),#2079,.F.);
#15067=ADVANCED_FACE('',(#3087),#2080,.F.);
#15068=ADVANCED_FACE('',(#3088),#2081,.F.);
#15069=ADVANCED_FACE('',(#3089),#2082,.F.);
#15070=ADVANCED_FACE('',(#3090),#2083,.F.);
#15071=ADVANCED_FACE('',(#3091),#2084,.F.);
#15072=ADVANCED_FACE('',(#3092),#2085,.F.);
#15073=ADVANCED_FACE('',(#3093),#2086,.F.);
#15074=ADVANCED_FACE('',(#3094),#2087,.F.);
#15075=ADVANCED_FACE('',(#3095),#2088,.F.);
#15076=ADVANCED_FACE('',(#3096),#2089,.F.);
#15077=ADVANCED_FACE('',(#3097),#2090,.F.);
#15078=ADVANCED_FACE('',(#3098),#2091,.F.);
#15079=ADVANCED_FACE('',(#3099),#2092,.F.);
#15080=ADVANCED_FACE('',(#3100),#2093,.F.);
#15081=ADVANCED_FACE('',(#3101),#2094,.F.);
#15082=ADVANCED_FACE('',(#3102),#2095,.F.);
#15083=ADVANCED_FACE('',(#3103),#2096,.T.);
#15084=ADVANCED_FACE('',(#3104,#1661),#14554,.F.);
#15085=ADVANCED_FACE('',(#3105,#1662),#14555,.F.);
#15086=ADVANCED_FACE('',(#3106),#2097,.T.);
#15087=ADVANCED_FACE('',(#3107),#14556,.F.);
#15088=ADVANCED_FACE('',(#3108),#14557,.F.);
#15089=ADVANCED_FACE('',(#3109),#14558,.F.);
#15090=ADVANCED_FACE('',(#3110),#14559,.F.);
#15091=ADVANCED_FACE('',(#3111,#1663),#14560,.T.);
#15092=ADVANCED_FACE('',(#3112),#258,.F.);
#15093=ADVANCED_FACE('',(#3113),#2098,.F.);
#15094=ADVANCED_FACE('',(#3114),#259,.F.);
#15095=ADVANCED_FACE('',(#3115),#14561,.F.);
#15096=ADVANCED_FACE('',(#3116),#2099,.F.);
#15097=ADVANCED_FACE('',(#3117),#14562,.F.);
#15098=ADVANCED_FACE('',(#3118),#2100,.F.);
#15099=ADVANCED_FACE('',(#3119),#14563,.F.);
#15100=ADVANCED_FACE('',(#3120),#2101,.T.);
#15101=ADVANCED_FACE('',(#3121),#14564,.T.);
#15102=ADVANCED_FACE('',(#3122,#1664),#14565,.T.);
#15103=ADVANCED_FACE('',(#3123,#1665),#14566,.F.);
#15104=ADVANCED_FACE('',(#3124),#2102,.T.);
#15105=ADVANCED_FACE('',(#3125),#2103,.T.);
#15106=ADVANCED_FACE('',(#3126,#1666),#14567,.T.);
#15107=ADVANCED_FACE('',(#3127,#1667),#2104,.T.);
#15108=ADVANCED_FACE('',(#3128,#1668),#14568,.F.);
#15109=ADVANCED_FACE('',(#3129),#2105,.T.);
#15480=CLOSED_SHELL('',(#15047,#15048,#15049,#15050,#15051,#15052,#15053,
#15054,#15055,#15056,#15057,#15058,#15059,#15060,#15061,#15062,#15063,#15064,
#15065,#15066,#15067,#15068,#15069,#15070,#15071,#15072,#15073,#15074,#15075,
#15076,#15077,#15078,#15079,#15080,#15081,#15082,#15083,#15084,#15085,#15086,
#15087,#15088,#15089,#15090,#15091,#15092,#15093,#15094,#15095,#15096,#15097,
#15098,#15099,#15100,#15101,#15102,#15103,#15104,#15105,#15106,#15107,#15108,
#15109));
#16184=AXIS2_PLACEMENT_3D('',#44079,#18213,#18214);
#16185=AXIS2_PLACEMENT_3D('',#44080,#18215,#18216);
#16186=AXIS2_PLACEMENT_3D('',#44090,#18218,#18219);
#16187=AXIS2_PLACEMENT_3D('',#44092,#18220,#18221);
#16188=AXIS2_PLACEMENT_3D('',#44103,#18222,#18223);
#16189=AXIS2_PLACEMENT_3D('',#44154,#18225,#18226);
#16190=AXIS2_PLACEMENT_3D('',#44205,#18228,#18229);
#16191=AXIS2_PLACEMENT_3D('',#44253,#18231,#18232);
#16192=AXIS2_PLACEMENT_3D('',#44304,#18234,#18235);
#16193=AXIS2_PLACEMENT_3D('',#44355,#18237,#18238);
#16194=AXIS2_PLACEMENT_3D('',#44403,#18240,#18241);
#16195=AXIS2_PLACEMENT_3D('',#44454,#18243,#18244);
#16196=AXIS2_PLACEMENT_3D('',#44505,#18246,#18247);
#16197=AXIS2_PLACEMENT_3D('',#44553,#18249,#18250);
#16198=AXIS2_PLACEMENT_3D('',#44604,#18252,#18253);
#16199=AXIS2_PLACEMENT_3D('',#44652,#18255,#18256);
#16200=AXIS2_PLACEMENT_3D('',#44703,#18258,#18259);
#16201=AXIS2_PLACEMENT_3D('',#44754,#18261,#18262);
#16202=AXIS2_PLACEMENT_3D('',#44802,#18264,#18265);
#16203=AXIS2_PLACEMENT_3D('',#44853,#18267,#18268);
#16204=AXIS2_PLACEMENT_3D('',#44904,#18270,#18271);
#16205=AXIS2_PLACEMENT_3D('',#44958,#18273,#18274);
#16206=AXIS2_PLACEMENT_3D('',#44972,#18276,#18277);
#16207=AXIS2_PLACEMENT_3D('',#44974,#18278,#18279);
#16208=AXIS2_PLACEMENT_3D('',#44984,#18280,#18281);
#16209=AXIS2_PLACEMENT_3D('',#45008,#18283,#18284);
#16210=AXIS2_PLACEMENT_3D('',#45033,#18286,#18287);
#16211=AXIS2_PLACEMENT_3D('',#45058,#18289,#18290);
#16212=AXIS2_PLACEMENT_3D('',#45082,#18292,#18293);
#16213=AXIS2_PLACEMENT_3D('',#45107,#18295,#18296);
#16214=AXIS2_PLACEMENT_3D('',#45132,#18298,#18299);
#16215=AXIS2_PLACEMENT_3D('',#45156,#18301,#18302);
#16216=AXIS2_PLACEMENT_3D('',#45181,#18304,#18305);
#16217=AXIS2_PLACEMENT_3D('',#45206,#18307,#18308);
#16218=AXIS2_PLACEMENT_3D('',#45230,#18310,#18311);
#16219=AXIS2_PLACEMENT_3D('',#45254,#18313,#18314);
#16220=AXIS2_PLACEMENT_3D('',#45280,#18316,#18317);
#16221=AXIS2_PLACEMENT_3D('',#45304,#18319,#18320);
#16222=AXIS2_PLACEMENT_3D('',#45328,#18322,#18323);
#16223=AXIS2_PLACEMENT_3D('',#45354,#18325,#18326);
#16224=AXIS2_PLACEMENT_3D('',#45378,#18328,#18329);
#16225=AXIS2_PLACEMENT_3D('',#45409,#18331,#18332);
#16226=AXIS2_PLACEMENT_3D('',#45411,#18333,#18334);
#16227=AXIS2_PLACEMENT_3D('',#45414,#18336,#18337);
#16228=AXIS2_PLACEMENT_3D('',#45415,#18338,#18339);
#16229=AXIS2_PLACEMENT_3D('',#45417,#18340,#18341);
#16230=AXIS2_PLACEMENT_3D('',#45418,#18342,#18343);
#16231=AXIS2_PLACEMENT_3D('',#45420,#18344,#18345);
#16232=AXIS2_PLACEMENT_3D('',#45421,#18346,#18347);
#16233=AXIS2_PLACEMENT_3D('',#45423,#18348,#18349);
#16234=AXIS2_PLACEMENT_3D('',#45425,#18351,#18352);
#16235=AXIS2_PLACEMENT_3D('',#45434,#18357,#18358);
#16236=AXIS2_PLACEMENT_3D('',#45440,#18362,#18363);
#16237=AXIS2_PLACEMENT_3D('',#45442,#18364,#18365);
#16238=AXIS2_PLACEMENT_3D('',#45444,#18367,#18368);
#16239=AXIS2_PLACEMENT_3D('',#45448,#18371,#18372);
#16240=AXIS2_PLACEMENT_3D('',#45450,#18373,#18374);
#16241=AXIS2_PLACEMENT_3D('',#45451,#18375,#18376);
#16242=AXIS2_PLACEMENT_3D('',#46060,#18377,#18378);
#16243=AXIS2_PLACEMENT_3D('',#46711,#18379,#18380);
#16244=AXIS2_PLACEMENT_3D('',#46713,#18382,#18383);
#16245=AXIS2_PLACEMENT_3D('',#46714,#18384,#18385);
#16246=AXIS2_PLACEMENT_3D('',#46716,#18387,#18388);
#16247=AXIS2_PLACEMENT_3D('',#46718,#18389,#18390);
#16248=AXIS2_PLACEMENT_3D('',#46722,#18393,#18394);
#16249=AXIS2_PLACEMENT_3D('',#46723,#18395,#18396);
#16250=AXIS2_PLACEMENT_3D('',#46724,#18397,#18398);
#16251=AXIS2_PLACEMENT_3D('',#46726,#18399,#18400);
#16252=AXIS2_PLACEMENT_3D('',#46728,#18402,#18403);
#16253=AXIS2_PLACEMENT_3D('',#46729,#18404,#18405);
#16254=AXIS2_PLACEMENT_3D('',#46731,#18406,#18407);
#16255=AXIS2_PLACEMENT_3D('',#46733,#18408,#18409);
#16256=AXIS2_PLACEMENT_3D('',#46734,#18410,#18411);
#16257=AXIS2_PLACEMENT_3D('',#46736,#18412,#18413);
#16258=AXIS2_PLACEMENT_3D('',#46738,#18414,#18415);
#16259=AXIS2_PLACEMENT_3D('',#46739,#18416,#18417);
#16260=AXIS2_PLACEMENT_3D('',#46741,#18419,#18420);
#16261=AXIS2_PLACEMENT_3D('',#46744,#18422,#18423);
#16262=AXIS2_PLACEMENT_3D('',#46745,#18424,#18425);
#16263=AXIS2_PLACEMENT_3D('',#46747,#18426,#18427);
#16264=AXIS2_PLACEMENT_3D('',#46748,#18428,#18429);
#16265=AXIS2_PLACEMENT_3D('',#46751,#18431,#18432);
#16266=AXIS2_PLACEMENT_3D('',#46752,#18433,#18434);
#16267=AXIS2_PLACEMENT_3D('',#46753,#18435,#18436);
#18213=DIRECTION('axis',(0.,0.,1.));
#18214=DIRECTION('refdir',(1.,0.,0.));
#18215=DIRECTION('center_axis',(-1.,0.,0.));
#18216=DIRECTION('ref_axis',(0.,-0.346908023969935,0.937899153910096));
#18217=DIRECTION('',(-1.,0.,0.));
#18218=DIRECTION('center_axis',(1.,0.,0.));
#18219=DIRECTION('ref_axis',(0.,1.,0.));
#18220=DIRECTION('center_axis',(1.,0.,0.));
#18221=DIRECTION('ref_axis',(0.,1.,0.));
#18222=DIRECTION('center_axis',(-1.,0.,0.));
#18223=DIRECTION('ref_axis',(0.,1.,0.));
#18224=DIRECTION('',(-1.,0.,0.));
#18225=DIRECTION('center_axis',(-1.,0.,0.));
#18226=DIRECTION('ref_axis',(0.,1.,0.));
#18227=DIRECTION('',(-1.,0.,0.));
#18228=DIRECTION('center_axis',(-1.,0.,0.));
#18229=DIRECTION('ref_axis',(0.,1.,0.));
#18230=DIRECTION('',(-1.,0.,0.));
#18231=DIRECTION('center_axis',(-1.,0.,0.));
#18232=DIRECTION('ref_axis',(0.,1.,0.));
#18233=DIRECTION('',(-1.,0.,0.));
#18234=DIRECTION('center_axis',(-1.,0.,0.));
#18235=DIRECTION('ref_axis',(0.,1.,0.));
#18236=DIRECTION('',(-1.,0.,0.));
#18237=DIRECTION('center_axis',(-1.,0.,0.));
#18238=DIRECTION('ref_axis',(0.,1.,0.));
#18239=DIRECTION('',(-1.,0.,0.));
#18240=DIRECTION('center_axis',(-1.,0.,0.));
#18241=DIRECTION('ref_axis',(0.,1.,0.));
#18242=DIRECTION('',(-1.,0.,0.));
#18243=DIRECTION('center_axis',(-1.,0.,0.));
#18244=DIRECTION('ref_axis',(0.,1.,0.));
#18245=DIRECTION('',(-1.,0.,0.));
#18246=DIRECTION('center_axis',(-1.,0.,0.));
#18247=DIRECTION('ref_axis',(0.,1.,0.));
#18248=DIRECTION('',(-1.,0.,0.));
#18249=DIRECTION('center_axis',(-1.,0.,0.));
#18250=DIRECTION('ref_axis',(0.,1.,0.));
#18251=DIRECTION('',(-1.,0.,0.));
#18252=DIRECTION('center_axis',(-1.,0.,0.));
#18253=DIRECTION('ref_axis',(0.,1.,0.));
#18254=DIRECTION('',(-1.,0.,0.));
#18255=DIRECTION('center_axis',(-1.,0.,0.));
#18256=DIRECTION('ref_axis',(0.,1.,0.));
#18257=DIRECTION('',(-1.,0.,0.));
#18258=DIRECTION('center_axis',(-1.,0.,0.));
#18259=DIRECTION('ref_axis',(0.,1.,0.));
#18260=DIRECTION('',(-1.,0.,0.));
#18261=DIRECTION('center_axis',(-1.,0.,0.));
#18262=DIRECTION('ref_axis',(0.,1.,0.));
#18263=DIRECTION('',(-1.,0.,0.));
#18264=DIRECTION('center_axis',(-1.,0.,0.));
#18265=DIRECTION('ref_axis',(0.,1.,0.));
#18266=DIRECTION('',(-1.,0.,0.));
#18267=DIRECTION('center_axis',(-1.,0.,0.));
#18268=DIRECTION('ref_axis',(0.,1.,0.));
#18269=DIRECTION('',(-1.,0.,0.));
#18270=DIRECTION('center_axis',(-1.,0.,0.));
#18271=DIRECTION('ref_axis',(0.,0.887282355496419,-0.461226648866614));
#18272=DIRECTION('',(-1.,0.,0.));
#18273=DIRECTION('center_axis',(-1.,0.,0.));
#18274=DIRECTION('ref_axis',(0.,1.,-1.07644854835951E-13));
#18275=DIRECTION('',(-1.,1.22464679914735E-16,-1.31976902897796E-29));
#18276=DIRECTION('center_axis',(1.,0.,0.));
#18277=DIRECTION('ref_axis',(0.,1.,-1.07644854835951E-13));
#18278=DIRECTION('center_axis',(1.,0.,0.));
#18279=DIRECTION('ref_axis',(0.,1.,-1.07644854835951E-13));
#18280=DIRECTION('center_axis',(-1.,0.,0.));
#18281=DIRECTION('ref_axis',(0.,1.,-1.07644854835951E-13));
#18282=DIRECTION('',(-1.,1.22464679914735E-16,-1.31976902897796E-29));
#18283=DIRECTION('center_axis',(-1.,0.,0.));
#18284=DIRECTION('ref_axis',(0.,1.,-1.07644854835951E-13));
#18285=DIRECTION('',(-1.,1.22464679914735E-16,-1.31976902897796E-29));
#18286=DIRECTION('center_axis',(-1.,0.,0.));
#18287=DIRECTION('ref_axis',(0.,1.,-1.07644854835951E-13));
#18288=DIRECTION('',(-1.,1.22464679914735E-16,-1.31976902897796E-29));
#18289=DIRECTION('center_axis',(-1.,0.,0.));
#18290=DIRECTION('ref_axis',(0.,1.,-1.07644854835951E-13));
#18291=DIRECTION('',(-1.,1.22464679914735E-16,-1.31976902897796E-29));
#18292=DIRECTION('center_axis',(-1.,0.,0.));
#18293=DIRECTION('ref_axis',(0.,1.,-1.07644854835951E-13));
#18294=DIRECTION('',(-1.,1.22464679914735E-16,-1.31976902897796E-29));
#18295=DIRECTION('center_axis',(-1.,0.,0.));
#18296=DIRECTION('ref_axis',(0.,1.,-1.07644854835951E-13));
#18297=DIRECTION('',(-1.,1.22464679914735E-16,-1.31976902897796E-29));
#18298=DIRECTION('center_axis',(-1.,0.,0.));
#18299=DIRECTION('ref_axis',(0.,1.,-1.07644854835951E-13));
#18300=DIRECTION('',(-1.,1.22464679914735E-16,-1.31976902897796E-29));
#18301=DIRECTION('center_axis',(-1.,0.,0.));
#18302=DIRECTION('ref_axis',(0.,1.,-1.07644854835951E-13));
#18303=DIRECTION('',(-1.,1.22464679914735E-16,-1.31976902897796E-29));
#18304=DIRECTION('center_axis',(-1.,0.,0.));
#18305=DIRECTION('ref_axis',(0.,1.,-1.07644854835951E-13));
#18306=DIRECTION('',(-1.,1.22464679914735E-16,-1.31976902897796E-29));
#18307=DIRECTION('center_axis',(-1.,0.,0.));
#18308=DIRECTION('ref_axis',(0.,1.,-1.07644854835951E-13));
#18309=DIRECTION('',(-1.,1.22464679914735E-16,-1.31976902897796E-29));
#18310=DIRECTION('center_axis',(-1.,0.,0.));
#18311=DIRECTION('ref_axis',(0.,1.,-1.07644854835951E-13));
#18312=DIRECTION('',(-1.,1.22464679914735E-16,-1.31976902897796E-29));
#18313=DIRECTION('center_axis',(-1.,0.,0.));
#18314=DIRECTION('ref_axis',(0.,1.,-1.07644854835951E-13));
#18315=DIRECTION('',(-1.,1.22464679914735E-16,-1.31976902897796E-29));
#18316=DIRECTION('center_axis',(-1.,0.,0.));
#18317=DIRECTION('ref_axis',(0.,1.,-1.07644854835951E-13));
#18318=DIRECTION('',(-1.,1.22464679914735E-16,-1.31976902897796E-29));
#18319=DIRECTION('center_axis',(-1.,0.,0.));
#18320=DIRECTION('ref_axis',(0.,1.,-1.07644854835951E-13));
#18321=DIRECTION('',(-1.,1.22464679914735E-16,-1.31976902897796E-29));
#18322=DIRECTION('center_axis',(-1.,0.,0.));
#18323=DIRECTION('ref_axis',(0.,1.,-1.07644854835951E-13));
#18324=DIRECTION('',(-1.,1.22464679914735E-16,-1.31976902897796E-29));
#18325=DIRECTION('center_axis',(-1.,0.,0.));
#18326=DIRECTION('ref_axis',(0.,1.,-1.07644854835951E-13));
#18327=DIRECTION('',(-1.,1.22464679914735E-16,-1.31976902897796E-29));
#18328=DIRECTION('center_axis',(-1.,0.,0.));
#18329=DIRECTION('ref_axis',(0.,-0.628210160162024,-0.778043697146377));
#18330=DIRECTION('',(-1.,1.22464679914735E-16,-1.31976902897796E-29));
#18331=DIRECTION('center_axis',(0.,0.,1.));
#18332=DIRECTION('ref_axis',(1.,0.,0.));
#18333=DIRECTION('center_axis',(0.,0.,1.));
#18334=DIRECTION('ref_axis',(1.,0.,0.));
#18335=DIRECTION('',(0.,0.,1.));
#18336=DIRECTION('center_axis',(0.,0.,1.));
#18337=DIRECTION('ref_axis',(1.,0.,0.));
#18338=DIRECTION('center_axis',(0.,0.,-1.));
#18339=DIRECTION('ref_axis',(-1.,0.,0.));
#18340=DIRECTION('center_axis',(0.,0.,-1.));
#18341=DIRECTION('ref_axis',(1.,0.,0.));
#18342=DIRECTION('center_axis',(0.,0.,1.));
#18343=DIRECTION('ref_axis',(1.,0.,0.));
#18344=DIRECTION('center_axis',(0.,0.,1.));
#18345=DIRECTION('ref_axis',(1.,0.,0.));
#18346=DIRECTION('center_axis',(0.,0.,1.));
#18347=DIRECTION('ref_axis',(1.,0.,0.));
#18348=DIRECTION('center_axis',(0.,0.,1.));
#18349=DIRECTION('ref_axis',(1.,0.,0.));
#18350=DIRECTION('',(0.,0.,-1.));
#18351=DIRECTION('center_axis',(0.,-1.,0.));
#18352=DIRECTION('ref_axis',(0.,0.,-1.));
#18353=DIRECTION('',(0.,0.,1.));
#18354=DIRECTION('',(1.,0.,0.));
#18355=DIRECTION('',(0.,0.,-1.));
#18356=DIRECTION('',(-1.,0.,0.));
#18357=DIRECTION('center_axis',(-1.,0.,0.));
#18358=DIRECTION('ref_axis',(0.,0.,1.));
#18359=DIRECTION('',(0.,-1.,0.));
#18360=DIRECTION('',(0.,1.,0.));
#18361=DIRECTION('',(0.,0.,1.));
#18362=DIRECTION('center_axis',(0.,0.,1.));
#18363=DIRECTION('ref_axis',(1.,0.,0.));
#18364=DIRECTION('center_axis',(0.,0.,1.));
#18365=DIRECTION('ref_axis',(1.,0.,0.));
#18366=DIRECTION('',(1.,0.,0.));
#18367=DIRECTION('center_axis',(0.,1.,0.));
#18368=DIRECTION('ref_axis',(0.,0.,1.));
#18369=DIRECTION('',(0.,0.,-1.));
#18370=DIRECTION('',(-1.,0.,0.));
#18371=DIRECTION('center_axis',(0.,0.,1.));
#18372=DIRECTION('ref_axis',(1.,0.,0.));
#18373=DIRECTION('center_axis',(0.,0.,-1.));
#18374=DIRECTION('ref_axis',(1.,0.,0.));
#18375=DIRECTION('center_axis',(0.,0.,-1.));
#18376=DIRECTION('ref_axis',(1.,0.,0.));
#18377=DIRECTION('center_axis',(-1.,0.,0.));
#18378=DIRECTION('ref_axis',(0.,1.,-1.07644854835951E-13));
#18379=DIRECTION('center_axis',(-1.,0.,0.));
#18380=DIRECTION('ref_axis',(0.,1.,0.));
#18381=DIRECTION('',(0.,0.,-1.));
#18382=DIRECTION('center_axis',(-1.,0.,0.));
#18383=DIRECTION('ref_axis',(0.,1.,0.));
#18384=DIRECTION('center_axis',(-1.,0.,0.));
#18385=DIRECTION('ref_axis',(0.,1.,0.));
#18386=DIRECTION('',(0.,0.,-1.));
#18387=DIRECTION('center_axis',(0.,0.,1.));
#18388=DIRECTION('ref_axis',(-1.,0.,0.));
#18389=DIRECTION('center_axis',(0.,0.,1.));
#18390=DIRECTION('ref_axis',(-1.,0.,0.));
#18391=DIRECTION('',(0.,0.,1.));
#18392=DIRECTION('',(0.,0.,1.));
#18393=DIRECTION('center_axis',(0.,0.,1.));
#18394=DIRECTION('ref_axis',(-1.,0.,0.));
#18395=DIRECTION('center_axis',(0.,0.,1.));
#18396=DIRECTION('ref_axis',(-1.,0.,0.));
#18397=DIRECTION('center_axis',(0.,0.,1.));
#18398=DIRECTION('ref_axis',(1.,0.,0.));
#18399=DIRECTION('center_axis',(0.,0.,1.));
#18400=DIRECTION('ref_axis',(1.,0.,0.));
#18401=DIRECTION('',(0.,0.,-1.));
#18402=DIRECTION('center_axis',(0.,0.,1.));
#18403=DIRECTION('ref_axis',(1.,0.,0.));
#18404=DIRECTION('center_axis',(0.,0.,1.));
#18405=DIRECTION('ref_axis',(1.,0.,0.));
#18406=DIRECTION('center_axis',(0.,0.,1.));
#18407=DIRECTION('ref_axis',(1.,0.,0.));
#18408=DIRECTION('center_axis',(0.,0.,1.));
#18409=DIRECTION('ref_axis',(1.,0.,0.));
#18410=DIRECTION('center_axis',(0.,0.,1.));
#18411=DIRECTION('ref_axis',(1.,0.,0.));
#18412=DIRECTION('center_axis',(0.,0.,1.));
#18413=DIRECTION('ref_axis',(1.,0.,0.));
#18414=DIRECTION('center_axis',(0.,0.,-1.));
#18415=DIRECTION('ref_axis',(1.,0.,0.));
#18416=DIRECTION('center_axis',(0.,0.,1.));
#18417=DIRECTION('ref_axis',(1.,0.,0.));
#18418=DIRECTION('',(0.,0.,-1.));
#18419=DIRECTION('center_axis',(0.,0.,1.));
#18420=DIRECTION('ref_axis',(1.,0.,0.));
#18421=DIRECTION('',(0.,0.,-1.));
#18422=DIRECTION('center_axis',(0.,0.,1.));
#18423=DIRECTION('ref_axis',(1.,0.,0.));
#18424=DIRECTION('center_axis',(0.,0.,1.));
#18425=DIRECTION('ref_axis',(1.,0.,0.));
#18426=DIRECTION('center_axis',(0.,0.,1.));
#18427=DIRECTION('ref_axis',(1.,0.,0.));
#18428=DIRECTION('center_axis',(0.,0.,1.));
#18429=DIRECTION('ref_axis',(1.,0.,0.));
#18430=DIRECTION('',(0.,0.,-1.));
#18431=DIRECTION('center_axis',(0.,0.,1.));
#18432=DIRECTION('ref_axis',(1.,0.,0.));
#18433=DIRECTION('center_axis',(0.,0.,1.));
#18434=DIRECTION('ref_axis',(1.,0.,0.));
#18435=DIRECTION('center_axis',(0.,0.,1.));
#18436=DIRECTION('ref_axis',(1.,0.,0.));
#18437=DIRECTION('',(0.,0.,-1.));
#44079=CARTESIAN_POINT('',(0.,0.,0.));
#44080=CARTESIAN_POINT('Origin',(17.,0.,10.));
#44081=CARTESIAN_POINT('',(8.38741669750802,-2.51341528648493,10.0004125898919));
#44082=CARTESIAN_POINT('',(8.11258330249198,-2.51593117465217,9.99678855536978));
#44083=CARTESIAN_POINT('',(17.,-2.5175,10.));
#44084=CARTESIAN_POINT('',(8.,-1.91346599666512,11.6359872033749));
#44085=CARTESIAN_POINT('Ctrl Pts',(8.11258330249198,-2.51593117465217,9.99678855536978));
#44086=CARTESIAN_POINT('Ctrl Pts',(8.07505553499465,-2.5106778598197,10.5892880216948));
#44087=CARTESIAN_POINT('Ctrl Pts',(8.03752776749733,-2.29922182808408,11.1848035603043));
#44088=CARTESIAN_POINT('Ctrl Pts',(8.,-1.91346599666512,11.6359872033749));
#44089=CARTESIAN_POINT('',(8.,0.,12.5175));
#44090=CARTESIAN_POINT('Origin',(8.,0.,10.));
#44091=CARTESIAN_POINT('',(8.,1.91705370942339,11.63867864773));
#44092=CARTESIAN_POINT('Origin',(8.,0.,10.));
#44093=CARTESIAN_POINT('Ctrl Pts',(8.,1.91705735205381,11.6386813803727));
#44094=CARTESIAN_POINT('Ctrl Pts',(8.05125205967898,1.39129213527502,12.2512665672672));
#44095=CARTESIAN_POINT('Ctrl Pts',(8.10250411935795,0.544371212086402,12.59099264795));
#44096=CARTESIAN_POINT('Ctrl Pts',(8.15375617903693,-0.258560825221013,
12.5080805624475));
#44097=CARTESIAN_POINT('Ctrl Pts',(8.20650761555986,-1.08498260540997,12.4227428873811));
#44098=CARTESIAN_POINT('Ctrl Pts',(8.25925905208279,-1.86480406571553,11.8896768067268));
#44099=CARTESIAN_POINT('Ctrl Pts',(8.31201048860571,-2.2437397594872,11.1506185698235));
#44100=CARTESIAN_POINT('Ctrl Pts',(8.33714589157315,-2.4242979013978,10.7984665181368));
#44101=CARTESIAN_POINT('Ctrl Pts',(8.36228129454058,-2.51383878282056,10.3995459271082));
#44102=CARTESIAN_POINT('Ctrl Pts',(8.38741669750802,-2.51341528648493,10.0004125898919));
#44103=CARTESIAN_POINT('Origin',(17.,0.,10.));
#44104=CARTESIAN_POINT('',(9.38741669750802,-2.51821640390817,9.99779587498902));
#44105=CARTESIAN_POINT('',(9.11258330249198,-2.52124832125375,10.0007652502423));
#44106=CARTESIAN_POINT('',(17.,-2.5175,10.));
#44107=CARTESIAN_POINT('Ctrl Pts',(9.11258330249198,-2.52124832125375,10.0007652502423));
#44108=CARTESIAN_POINT('Ctrl Pts',(9.10992719234634,-2.52141294296029,10.0426045038361));
#44109=CARTESIAN_POINT('Ctrl Pts',(9.1072710822007,-2.5204604246002,10.0844359799301));
#44110=CARTESIAN_POINT('Ctrl Pts',(9.10461497205506,-2.51836711132594,10.1262101550091));
#44111=CARTESIAN_POINT('Ctrl Pts',(9.05201425910005,-2.47691183852974,10.953491883468));
#44112=CARTESIAN_POINT('Ctrl Pts',(8.99941354614505,-1.98805378788741,11.7583010071421));
#44113=CARTESIAN_POINT('Ctrl Pts',(8.94681283319005,-1.27303790376294,12.1765352372871));
#44114=CARTESIAN_POINT('Ctrl Pts',(8.89421212023505,-0.558022019638478,
12.5947694674322));
#44115=CARTESIAN_POINT('Ctrl Pts',(8.84161140728004,0.383151697968126,12.6264288040482));
#44116=CARTESIAN_POINT('Ctrl Pts',(8.78901069432504,1.12455068265491,12.2569425195909));
#44117=CARTESIAN_POINT('Ctrl Pts',(8.73640998137004,1.8659496673417,11.8874562351336));
#44118=CARTESIAN_POINT('Ctrl Pts',(8.68380926841503,2.40757391910867,11.116824329603));
#44119=CARTESIAN_POINT('Ctrl Pts',(8.63120855546003,2.50428468514339,10.2942760189482));
#44120=CARTESIAN_POINT('Ctrl Pts',(8.57860784250503,2.60099545117811,9.47172770829336));
#44121=CARTESIAN_POINT('Ctrl Pts',(8.52600712955003,2.25279273148057,8.59726299251438));
#44122=CARTESIAN_POINT('Ctrl Pts',(8.47340641659503,1.61729847184723,8.06572620427011));
#44123=CARTESIAN_POINT('Ctrl Pts',(8.42080570364003,0.981804212213907,7.53418941602586));
#44124=CARTESIAN_POINT('Ctrl Pts',(8.36820499068502,0.0590184126448082,
7.34558055531628));
#44125=CARTESIAN_POINT('Ctrl Pts',(8.31560427773002,-0.733527071137423,
7.58705948364037));
#44126=CARTESIAN_POINT('Ctrl Pts',(8.26300356477502,-1.52607255491969,7.82853841196447));
#44127=CARTESIAN_POINT('Ctrl Pts',(8.21040285182001,-2.18837772291507,8.50010512932227));
#44128=CARTESIAN_POINT('Ctrl Pts',(8.15780213886501,-2.42039953698568,9.29386718638688));
#44129=CARTESIAN_POINT('Ctrl Pts',(8.14272919340733,-2.48688631923651,9.52132289031894));
#44130=CARTESIAN_POINT('Ctrl Pts',(8.12765624794966,-2.51804115702582,9.75881244500678));
#44131=CARTESIAN_POINT('Ctrl Pts',(8.11258330249198,-2.51593117465217,9.99678855536978));
#44132=CARTESIAN_POINT('Ctrl Pts',(8.38741669750802,-2.51341528648493,10.0004125898919));
#44133=CARTESIAN_POINT('Ctrl Pts',(8.41503273106351,-2.51294999499824,9.56188850305078));
#44134=CARTESIAN_POINT('Ctrl Pts',(8.442648764619,-2.40388679040722,9.12310760576339));
#44135=CARTESIAN_POINT('Ctrl Pts',(8.4702647981745,-2.1876220614921,8.74581465401795));
#44136=CARTESIAN_POINT('Ctrl Pts',(8.52301623469742,-1.77451874248758,8.0251193682683));
#44137=CARTESIAN_POINT('Ctrl Pts',(8.57576767122035,-0.970262177240812,
7.5287791899215));
#44138=CARTESIAN_POINT('Ctrl Pts',(8.62851910774328,-0.1408761191083,7.48239314407354));
#44139=CARTESIAN_POINT('Ctrl Pts',(8.68127054426621,0.688509939024223,7.43600709822558));
#44140=CARTESIAN_POINT('Ctrl Pts',(8.73402198078914,1.54302549004246,7.8395751848765));
#44141=CARTESIAN_POINT('Ctrl Pts',(8.78677341731206,2.03398159212986,8.50960439185275));
#44142=CARTESIAN_POINT('Ctrl Pts',(8.83952485383499,2.52493769421725,9.179633598829));
#44143=CARTESIAN_POINT('Ctrl Pts',(8.89227629035792,2.65233434737381,10.1161239261306));
#44144=CARTESIAN_POINT('Ctrl Pts',(8.94502772688085,2.35817766113461,10.8929680036272));
#44145=CARTESIAN_POINT('Ctrl Pts',(8.99777916340378,2.0640209748954,11.6698120811238));
#44146=CARTESIAN_POINT('Ctrl Pts',(9.05053059992671,1.34831094926045,12.2870099088155));
#44147=CARTESIAN_POINT('Ctrl Pts',(9.10328203644964,0.536674424493379,12.4637998105904));
#44148=CARTESIAN_POINT('Ctrl Pts',(9.15603347297256,-0.274962100273664,
12.6405897123653));
#44149=CARTESIAN_POINT('Ctrl Pts',(9.20878490949549,-1.18252512417281,12.3769716882235));
#44150=CARTESIAN_POINT('Ctrl Pts',(9.26153634601842,-1.77313330145451,11.7928622005606));
#44151=CARTESIAN_POINT('Ctrl Pts',(9.30349646318162,-2.24292123425351,11.3282435256204));
#44152=CARTESIAN_POINT('Ctrl Pts',(9.34545658034482,-2.51216861793005,10.6608466481397));
#44153=CARTESIAN_POINT('Ctrl Pts',(9.38741669750802,-2.51821640390817,9.99779587498902));
#44154=CARTESIAN_POINT('Origin',(17.,0.,10.));
#44155=CARTESIAN_POINT('',(10.387416697508,-2.52029863869409,10.0015637155967));
#44156=CARTESIAN_POINT('',(10.112583302492,-2.51430853248195,10.001394303415));
#44157=CARTESIAN_POINT('',(17.,-2.5175,10.));
#44158=CARTESIAN_POINT('Ctrl Pts',(10.112583302492,-2.51430853248195,10.001394303415));
#44159=CARTESIAN_POINT('Ctrl Pts',(10.092198136743,-2.51595777248054,10.3247931866629));
#44160=CARTESIAN_POINT('Ctrl Pts',(10.0718129709941,-2.45799321307868,10.6476234550357));
#44161=CARTESIAN_POINT('Ctrl Pts',(10.0514278052451,-2.33765469185702,10.9452326133532));
#44162=CARTESIAN_POINT('Ctrl Pts',(9.9988270922901,-2.02714007107045,11.7131662226365));
#44163=CARTESIAN_POINT('Ctrl Pts',(9.9462263793351,-1.30132911626528,12.3131734369901));
#44164=CARTESIAN_POINT('Ctrl Pts',(9.8936256663801,-0.488698459628603,12.4737145429049));
#44165=CARTESIAN_POINT('Ctrl Pts',(9.84102495342509,0.323932197008068,12.6342556488198));
#44166=CARTESIAN_POINT('Ctrl Pts',(9.78842424047009,1.22338255547628,12.3553306462958));
#44167=CARTESIAN_POINT('Ctrl Pts',(9.73582352751509,1.80259317536673,11.7631664355228));
#44168=CARTESIAN_POINT('Ctrl Pts',(9.68322281456008,2.38180379525719,11.1710022247498));
#44169=CARTESIAN_POINT('Ctrl Pts',(9.63062210160508,2.64077467656993,10.2655988057278));
#44170=CARTESIAN_POINT('Ctrl Pts',(9.57802138865008,2.46230433720098,9.4567191109119));
#44171=CARTESIAN_POINT('Ctrl Pts',(9.52542067569508,2.28383399783203,8.64783941609604));
#44172=CARTESIAN_POINT('Ctrl Pts',(9.47281996274007,1.66792243778143,7.93548344548637));
#44173=CARTESIAN_POINT('Ctrl Pts',(9.42021924978507,0.893310282463933,7.64202084104588));
#44174=CARTESIAN_POINT('Ctrl Pts',(9.36761853683007,0.118698127146456,7.3485582366054));
#44175=CARTESIAN_POINT('Ctrl Pts',(9.31501782387507,-0.814614623437939,
7.47398899833411));
#44176=CARTESIAN_POINT('Ctrl Pts',(9.26241711092007,-1.48424475125507,7.96158154582029));
#44177=CARTESIAN_POINT('Ctrl Pts',(9.2124725081107,-2.12006143289624,8.42455276329856));
#44178=CARTESIAN_POINT('Ctrl Pts',(9.16252790530134,-2.51815282999178,9.2140339823356));
#44179=CARTESIAN_POINT('Ctrl Pts',(9.11258330249198,-2.52124832125375,10.0007652502423));
#44180=CARTESIAN_POINT('Ctrl Pts',(9.38741669750802,-2.51821640390817,9.99779587498902));
#44181=CARTESIAN_POINT('Ctrl Pts',(9.39820801686775,-2.51977177587378,9.82727221756083));
#44182=CARTESIAN_POINT('Ctrl Pts',(9.40899933622747,-2.5039186648545,9.65703601909512));
#44183=CARTESIAN_POINT('Ctrl Pts',(9.4197906555872,-2.46959121774327,9.4906105390579));
#44184=CARTESIAN_POINT('Ctrl Pts',(9.47254209211013,-2.30178762608609,8.67706931640221));
#44185=CARTESIAN_POINT('Ctrl Pts',(9.52529352863306,-1.69252711210748,7.95458782227486));
#44186=CARTESIAN_POINT('Ctrl Pts',(9.57804496515599,-0.918992044645595,
7.65185103954266));
#44187=CARTESIAN_POINT('Ctrl Pts',(9.63079640167891,-0.145456977183702,
7.34911425681047));
#44188=CARTESIAN_POINT('Ctrl Pts',(9.68354783820185,0.792352643761475,7.46612218547344));
#44189=CARTESIAN_POINT('Ctrl Pts',(9.73629927472478,1.46778672088276,7.94964481826351));
#44190=CARTESIAN_POINT('Ctrl Pts',(9.7890507112477,2.14322079800404,8.43316745105357));
#44191=CARTESIAN_POINT('Ctrl Pts',(9.84180214777063,2.55627933130144,9.2832047879707));
#44192=CARTESIAN_POINT('Ctrl Pts',(9.89455358429355,2.51904287005632,10.1130358196035));
#44193=CARTESIAN_POINT('Ctrl Pts',(9.94730502081648,2.4818064088112,10.9428668512363));
#44194=CARTESIAN_POINT('Ctrl Pts',(10.0000564573394,1.9942749530235,11.7524915775848));
#44195=CARTESIAN_POINT('Ctrl Pts',(10.0528078938623,1.27824867411093,12.1735761611315));
#44196=CARTESIAN_POINT('Ctrl Pts',(10.1055593303853,0.562222395198357,12.5946607446782));
#44197=CARTESIAN_POINT('Ctrl Pts',(10.1583107669082,-0.382298706839069,
12.6272051854231));
#44198=CARTESIAN_POINT('Ctrl Pts',(10.2110622034311,-1.12561003076715,12.2564032684892));
#44199=CARTESIAN_POINT('Ctrl Pts',(10.2638136399541,-1.86892135469524,11.8856013515554));
#44200=CARTESIAN_POINT('Ctrl Pts',(10.316565076477,-2.41102290051395,11.1114530769427));
#44201=CARTESIAN_POINT('Ctrl Pts',(10.3693165129999,-2.50528839198755,10.2861531872439));
#44202=CARTESIAN_POINT('Ctrl Pts',(10.3753499078359,-2.51606991694613,10.1917603058192));
#44203=CARTESIAN_POINT('Ctrl Pts',(10.381383302672,-2.52099311007268,10.0966982885981));
#44204=CARTESIAN_POINT('Ctrl Pts',(10.387416697508,-2.52029863869409,10.0015637155967));
#44205=CARTESIAN_POINT('Origin',(17.,0.,10.));
#44206=CARTESIAN_POINT('',(11.387416697508,-2.51373500251495,10.0008811020012));
#44207=CARTESIAN_POINT('',(11.112583302492,-2.51647995600113,9.99782029265504));
#44208=CARTESIAN_POINT('',(17.,-2.5175,10.));
#44209=CARTESIAN_POINT('Ctrl Pts',(11.112583302492,-2.51647995600113,9.99782029265504));
#44210=CARTESIAN_POINT('Ctrl Pts',(11.0744690811397,-2.51135536271962,10.601162700555));
#44211=CARTESIAN_POINT('Ctrl Pts',(11.0363548597874,-2.29335787087922,11.2078301743458));
#44212=CARTESIAN_POINT('Ctrl Pts',(10.9982406384351,-1.89829552552759,11.6596889786441));
#44213=CARTESIAN_POINT('Ctrl Pts',(10.9456399254801,-1.35307748643653,12.2832907319479));
#44214=CARTESIAN_POINT('Ctrl Pts',(10.8930392125251,-0.470617551500217,
12.612040242372));
#44215=CARTESIAN_POINT('Ctrl Pts',(10.8404384995701,0.349713918313006,12.4971570813192));
#44216=CARTESIAN_POINT('Ctrl Pts',(10.7878377866151,1.17004538812622,12.3822739202663));
#44217=CARTESIAN_POINT('Ctrl Pts',(10.7352370736601,1.92824839281636,11.8237580877364));
#44218=CARTESIAN_POINT('Ctrl Pts',(10.6826363607051,2.28118689753448,11.0743741314967));
#44219=CARTESIAN_POINT('Ctrl Pts',(10.6300356477501,2.63412540225261,10.3249901752571));
#44220=CARTESIAN_POINT('Ctrl Pts',(10.5774349347951,2.58179940699873,9.38473809530771));
#44221=CARTESIAN_POINT('Ctrl Pts',(10.5248342218401,2.14788981154851,8.67914312428277));
#44222=CARTESIAN_POINT('Ctrl Pts',(10.4722335088851,1.7139802160983,7.97354815325784));
#44223=CARTESIAN_POINT('Ctrl Pts',(10.4196327959301,0.89848702045178,7.50261029115733));
#44224=CARTESIAN_POINT('Ctrl Pts',(10.3670320829751,0.0704738041310564,
7.47945912120493));
#44225=CARTESIAN_POINT('Ctrl Pts',(10.3144313700201,-0.75753941218968,7.45630795125253));
#44226=CARTESIAN_POINT('Ctrl Pts',(10.2618306570651,-1.59807264918463,7.88094347344825));
#44227=CARTESIAN_POINT('Ctrl Pts',(10.2092299441101,-2.07073012429811,8.5611912366526));
#44228=CARTESIAN_POINT('Ctrl Pts',(10.1770143969041,-2.36021135651701,8.97781209017717));
#44229=CARTESIAN_POINT('Ctrl Pts',(10.144798849698,-2.51170216814413,9.49031324977247));
#44230=CARTESIAN_POINT('Ctrl Pts',(10.112583302492,-2.51430853248195,10.001394303415));
#44231=CARTESIAN_POINT('Ctrl Pts',(10.387416697508,-2.52029863869409,10.0015637155967));
#44232=CARTESIAN_POINT('Ctrl Pts',(10.4341347391949,-2.51492117812715,9.26491360929207));
#44233=CARTESIAN_POINT('Ctrl Pts',(10.4808527808818,-2.17272085367765,8.52391321726476));
#44234=CARTESIAN_POINT('Ctrl Pts',(10.5275708225687,-1.60543177741221,8.05553548493098));
#44235=CARTESIAN_POINT('Ctrl Pts',(10.5803222590916,-0.964880234234785,
7.52666917710177));
#44236=CARTESIAN_POINT('Ctrl Pts',(10.6330736956146,-0.0373477107514415,
7.34538806622821));
#44237=CARTESIAN_POINT('Ctrl Pts',(10.6858251321375,0.755189892849743,7.59416505899928));
#44238=CARTESIAN_POINT('Ctrl Pts',(10.7385765686604,1.54772749645094,7.84294205177034));
#44239=CARTESIAN_POINT('Ctrl Pts',(10.7913280051833,2.20527018016997,8.52177714818604));
#44240=CARTESIAN_POINT('Ctrl Pts',(10.8440794417063,2.42867242752584,9.32183795532995));
#44241=CARTESIAN_POINT('Ctrl Pts',(10.8968308782292,2.6520746748817,10.1218987624739));
#44242=CARTESIAN_POINT('Ctrl Pts',(10.9495823147521,2.44133648587441,11.043185280346));
#44243=CARTESIAN_POINT('Ctrl Pts',(11.0023337512751,1.89233207177004,11.6665631803213));
#44244=CARTESIAN_POINT('Ctrl Pts',(11.055085187798,1.34332765766567,12.2899410802967));
#44245=CARTESIAN_POINT('Ctrl Pts',(11.1078366243209,0.456057018464226,12.6154103623752));
#44246=CARTESIAN_POINT('Ctrl Pts',(11.1605880608438,-0.36582085049157,12.4949005236292));
#44247=CARTESIAN_POINT('Ctrl Pts',(11.2133394973668,-1.18769871944735,12.3743906848832));
#44248=CARTESIAN_POINT('Ctrl Pts',(11.2660909338897,-1.94418381815748,11.8079017253127));
#44249=CARTESIAN_POINT('Ctrl Pts',(11.3188423704126,-2.2911173230099,11.0531547493414));
#44250=CARTESIAN_POINT('Ctrl Pts',(11.3417004794444,-2.44144960594696,10.7261098420302));
#44251=CARTESIAN_POINT('Ctrl Pts',(11.3645585884762,-2.5148828983645,10.363716881786));
#44252=CARTESIAN_POINT('Ctrl Pts',(11.387416697508,-2.51373500251495,10.0008811020012));
#44253=CARTESIAN_POINT('Origin',(17.,0.,10.));
#44254=CARTESIAN_POINT('',(12.387416697508,-2.51713767377043,9.99773848900567));
#44255=CARTESIAN_POINT('',(12.112583302492,-2.52111941107521,10.0008984969629));
#44256=CARTESIAN_POINT('',(17.,-2.5175,10.));
#44257=CARTESIAN_POINT('Ctrl Pts',(12.112583302492,-2.52111941107521,10.0008984969629));
#44258=CARTESIAN_POINT('Ctrl Pts',(12.1093407384914,-2.52135655101894,10.0519832687507));
#44259=CARTESIAN_POINT('Ctrl Pts',(12.1060981744908,-2.51993661233261,10.1030546133874));
#44260=CARTESIAN_POINT('Ctrl Pts',(12.1028556104902,-2.51681755665027,10.1540219769643));
#44261=CARTESIAN_POINT('Ctrl Pts',(12.0502548975352,-2.46622038952963,10.9808120298638));
#44262=CARTESIAN_POINT('Ctrl Pts',(11.9976541845802,-1.96849772959592,11.7802392921331));
#44263=CARTESIAN_POINT('Ctrl Pts',(11.9450534716252,-1.24890136395571,12.1905110743009));
#44264=CARTESIAN_POINT('Ctrl Pts',(11.8924527586702,-0.52930499831549,12.6007828564687));
#44265=CARTESIAN_POINT('Ctrl Pts',(11.8398520457152,0.412165073031232,12.621899158535));
#44266=CARTESIAN_POINT('Ctrl Pts',(11.7872513327602,1.14943257671712,12.2443034851074));
#44267=CARTESIAN_POINT('Ctrl Pts',(11.7346506198052,1.886700080403,11.8667078116798));
#44268=CARTESIAN_POINT('Ctrl Pts',(11.6820499068502,2.41976501642805,11.0904001627582));
#44269=CARTESIAN_POINT('Ctrl Pts',(11.6294491938952,2.50738092542064,10.2667101008629));
#44270=CARTESIAN_POINT('Ctrl Pts',(11.5768484809402,2.59499683441322,9.44302003896762));
#44271=CARTESIAN_POINT('Ctrl Pts',(11.5242477679852,2.23716371637332,8.57194756409857));
#44272=CARTESIAN_POINT('Ctrl Pts',(11.4716470550302,1.59582426700453,8.04770947453438));
#44273=CARTESIAN_POINT('Ctrl Pts',(11.4190463420752,0.954484817635741,7.5234713849702));
#44274=CARTESIAN_POINT('Ctrl Pts',(11.3664456291202,0.0296390369380665,
7.34606768071088));
#44275=CARTESIAN_POINT('Ctrl Pts',(11.3138449161652,-0.760160371302549,
7.59578503800158));
#44276=CARTESIAN_POINT('Ctrl Pts',(11.2612442032102,-1.54995977954318,7.84550239529228));
#44277=CARTESIAN_POINT('Ctrl Pts',(11.2086434902552,-2.20471281532674,8.52234081413302));
#44278=CARTESIAN_POINT('Ctrl Pts',(11.1560427773002,-2.42810126159561,9.31998702164505));
#44279=CARTESIAN_POINT('Ctrl Pts',(11.1415562856974,-2.48962352373278,9.53966265792308));
#44280=CARTESIAN_POINT('Ctrl Pts',(11.1270697940947,-2.51842771657201,9.76850130316745));
#44281=CARTESIAN_POINT('Ctrl Pts',(11.112583302492,-2.51647995600113,9.99782029265504));
#44282=CARTESIAN_POINT('Ctrl Pts',(11.387416697508,-2.51373500251495,10.0008811020012));
#44283=CARTESIAN_POINT('Ctrl Pts',(11.4173100249991,-2.51223380980875,9.52637252495675));
#44284=CARTESIAN_POINT('Ctrl Pts',(11.4472033524903,-2.38317769596416,9.05110660128233));
#44285=CARTESIAN_POINT('Ctrl Pts',(11.4770966799814,-2.13175081935672,8.65315481349981));
#44286=CARTESIAN_POINT('Ctrl Pts',(11.5298481165043,-1.68806889985638,7.95090684600186));
#44287=CARTESIAN_POINT('Ctrl Pts',(11.5825995530273,-0.863323149861005,
7.48941590337823));
#44288=CARTESIAN_POINT('Ctrl Pts',(11.6353509895502,-0.0327272062512589,
7.47863480548892));
#44289=CARTESIAN_POINT('Ctrl Pts',(11.6881024260731,0.797868737358476,7.46785370759962));
#44290=CARTESIAN_POINT('Ctrl Pts',(11.740853862596,1.63431487458258,7.90778245444463));
#44291=CARTESIAN_POINT('Ctrl Pts',(11.793605299119,2.09607453959934,8.5982778314047));
#44292=CARTESIAN_POINT('Ctrl Pts',(11.8463567356419,2.5578342046161,9.28877320836478));
#44293=CARTESIAN_POINT('Ctrl Pts',(11.8991081721648,2.64490739742552,10.2298352154399));
#44294=CARTESIAN_POINT('Ctrl Pts',(11.9518596086878,2.31768063801954,10.9933327607025));
#44295=CARTESIAN_POINT('Ctrl Pts',(12.0046110452107,1.99045387861357,11.7568303059651));
#44296=CARTESIAN_POINT('Ctrl Pts',(12.0573624817336,1.24892716699225,12.3427633894151));
#44297=CARTESIAN_POINT('Ctrl Pts',(12.1101139182565,0.430454087136451,12.4845649100919));
#44298=CARTESIAN_POINT('Ctrl Pts',(12.1628653547795,-0.388018992719343,
12.6263664307688));
#44299=CARTESIAN_POINT('Ctrl Pts',(12.2156167913024,-1.28343844080961,12.3240363886725));
#44300=CARTESIAN_POINT('Ctrl Pts',(12.2683682278253,-1.84843800135739,11.7151182083536));
#44301=CARTESIAN_POINT('Ctrl Pts',(12.3080510510529,-2.27346486626798,11.2570530995647));
#44302=CARTESIAN_POINT('Ctrl Pts',(12.3477338742805,-2.51150847337059,10.6254910220656));
#44303=CARTESIAN_POINT('Ctrl Pts',(12.387416697508,-2.51713767377043,9.99773848900567));
#44304=CARTESIAN_POINT('Origin',(17.,0.,10.));
#44305=CARTESIAN_POINT('',(13.387416697508,-2.52103810132661,10.001041928985));
#44306=CARTESIAN_POINT('',(13.112583302492,-2.51415776047792,10.0012738589896));
#44307=CARTESIAN_POINT('',(17.,-2.5175,10.));
#44308=CARTESIAN_POINT('Ctrl Pts',(13.112583302492,-2.51415776047792,10.0012738589896));
#44309=CARTESIAN_POINT('Ctrl Pts',(13.0916116828881,-2.51570257838621,10.3340264679862));
#44310=CARTESIAN_POINT('Ctrl Pts',(13.0706400632842,-2.45424048782787,10.6662314315614));
#44311=CARTESIAN_POINT('Ctrl Pts',(13.0496684436802,-2.32706309090986,10.9710153210997));
#44312=CARTESIAN_POINT('Ctrl Pts',(12.9970677307252,-2.00807858346622,11.735469864416));
#44313=CARTESIAN_POINT('Ctrl Pts',(12.9444670177702,-1.27567943315398,12.3274185767768));
#44314=CARTESIAN_POINT('Ctrl Pts',(12.8918663048152,-0.461323760684686,
12.4789662705914));
#44315=CARTESIAN_POINT('Ctrl Pts',(12.8392655918602,0.353031911784589,12.6305139644061));
#44316=CARTESIAN_POINT('Ctrl Pts',(12.7866648789052,1.24934410641091,12.3416606396747));
#44317=CARTESIAN_POINT('Ctrl Pts',(12.7340641659502,1.82197341812958,11.7431311615882));
#44318=CARTESIAN_POINT('Ctrl Pts',(12.6814634529952,2.39460272984827,11.1446016835016));
#44319=CARTESIAN_POINT('Ctrl Pts',(12.6288627400402,2.64354915865928,10.2363960520598));
#44320=CARTESIAN_POINT('Ctrl Pts',(12.5762620270852,2.45614829825437,9.42953622388729));
#44321=CARTESIAN_POINT('Ctrl Pts',(12.5236613141302,2.26874743784946,8.62267639571484));
#44322=CARTESIAN_POINT('Ctrl Pts',(12.4710606011752,1.64499928822862,7.91716237081174));
#44323=CARTESIAN_POINT('Ctrl Pts',(12.4184598882202,0.867190344919238,7.63228500687628));
#44324=CARTESIAN_POINT('Ctrl Pts',(12.3658591752652,0.0893814016098554,
7.34740764294083));
#44325=CARTESIAN_POINT('Ctrl Pts',(12.3132584623102,-0.842488335388107,
7.48316693997303));
#44326=CARTESIAN_POINT('Ctrl Pts',(12.2606577493552,-1.50668736673329,7.97812301025402));
#44327=CARTESIAN_POINT('Ctrl Pts',(12.2112996004008,-2.12994193654405,8.4425675789753));
#44328=CARTESIAN_POINT('Ctrl Pts',(12.1619414514464,-2.51750967857237,9.22328862565574));
#44329=CARTESIAN_POINT('Ctrl Pts',(12.112583302492,-2.52111941107521,10.0008984969629));
#44330=CARTESIAN_POINT('Ctrl Pts',(12.387416697508,-2.51713767377043,9.99773848900567));
#44331=CARTESIAN_POINT('Ctrl Pts',(12.4004853108034,-2.5189915197724,9.79100281768763));
#44332=CARTESIAN_POINT('Ctrl Pts',(12.4135539240987,-2.49563861108269,9.58468031461302));
#44333=CARTESIAN_POINT('Ctrl Pts',(12.4266225373941,-2.44545626145838,9.38510392197382));
#44334=CARTESIAN_POINT('Ctrl Pts',(12.479373973917,-2.24289528800626,8.57951413445476));
#44335=CARTESIAN_POINT('Ctrl Pts',(12.53212541044,-1.60319366809675,7.88384087795828));
#44336=CARTESIAN_POINT('Ctrl Pts',(12.5848768469629,-0.817380208664749,
7.61457695408235));
#44337=CARTESIAN_POINT('Ctrl Pts',(12.6376282834858,-0.0315667492327322,
7.34531303020641));
#44338=CARTESIAN_POINT('Ctrl Pts',(12.6903797200088,0.900358549721807,7.50245843895104));
#44339=CARTESIAN_POINT('Ctrl Pts',(12.7431311565317,1.55442129220108,8.01452072288645));
#44340=CARTESIAN_POINT('Ctrl Pts',(12.7958825930546,2.20848403468036,8.52658300682186));
#44341=CARTESIAN_POINT('Ctrl Pts',(12.8486340295775,2.58468422068438,9.39356216594807));
#44342=CARTESIAN_POINT('Ctrl Pts',(12.9013854661005,2.51187160157225,10.2210307008325));
#44343=CARTESIAN_POINT('Ctrl Pts',(12.9541369026234,2.43905898246011,11.0484992357168));
#44344=CARTESIAN_POINT('Ctrl Pts',(13.0068883391463,1.91723355823185,11.8364571463594));
#44345=CARTESIAN_POINT('Ctrl Pts',(13.0596397756693,1.18379699541328,12.2264272247595));
#44346=CARTESIAN_POINT('Ctrl Pts',(13.1123912121922,0.450360432594741,12.6163973031597));
#44347=CARTESIAN_POINT('Ctrl Pts',(13.1651426487151,-0.494687268814085,
12.6083795493175));
#44348=CARTESIAN_POINT('Ctrl Pts',(13.217894085238,-1.2214017464924,12.206021597166));
#44349=CARTESIAN_POINT('Ctrl Pts',(13.270645521761,-1.94811622417074,11.8036636450145));
#44350=CARTESIAN_POINT('Ctrl Pts',(13.3233969582839,-2.45649747811857,11.0069654945536));
#44351=CARTESIAN_POINT('Ctrl Pts',(13.3761483948068,-2.51526019467618,10.1783806788171));
#44352=CARTESIAN_POINT('Ctrl Pts',(13.3799044957072,-2.51944432134875,10.119382320145));
#44353=CARTESIAN_POINT('Ctrl Pts',(13.3836605966076,-2.52134889274696,10.0602222968396));
#44354=CARTESIAN_POINT('Ctrl Pts',(13.387416697508,-2.52103810132661,10.001041928985));
#44355=CARTESIAN_POINT('Origin',(17.,0.,10.));
#44356=CARTESIAN_POINT('',(14.387416697508,-2.5142305845587,10.0013871638039));
#44357=CARTESIAN_POINT('',(14.112583302492,-2.51674334939835,9.9977931730102));
#44358=CARTESIAN_POINT('',(17.,-2.5175,10.));
#44359=CARTESIAN_POINT('Ctrl Pts',(14.112583302492,-2.51674334939835,9.9977931730102));
#44360=CARTESIAN_POINT('Ctrl Pts',(14.0738826272847,-2.51142956124591,10.6102558210133));
#44361=CARTESIAN_POINT('Ctrl Pts',(14.0351819520775,-2.28602139692528,11.2262225148951));
#44362=CARTESIAN_POINT('Ctrl Pts',(13.9964812768703,-1.87983305754009,11.6805716463953));
#44363=CARTESIAN_POINT('Ctrl Pts',(13.9438805639153,-1.32775493147994,12.2981083720319));
#44364=CARTESIAN_POINT('Ctrl Pts',(13.8912798509603,-0.441714862070872,
12.6170829616767));
#44365=CARTESIAN_POINT('Ctrl Pts',(13.8386791380053,0.377296548559049,12.4931387240453));
#44366=CARTESIAN_POINT('Ctrl Pts',(13.7860784250503,1.19630795918896,12.3691944864138));
#44367=CARTESIAN_POINT('Ctrl Pts',(13.7334777120953,1.94829071103973,11.8023314215061));
#44368=CARTESIAN_POINT('Ctrl Pts',(13.6808769991403,2.29292383346307,11.0490918343144));
#44369=CARTESIAN_POINT('Ctrl Pts',(13.6282762861853,2.63755695588642,10.2958522471228));
#44370=CARTESIAN_POINT('Ctrl Pts',(13.5756755732303,2.57484044888233,9.35623613764727));
#44371=CARTESIAN_POINT('Ctrl Pts',(13.5230748602753,2.13315759981582,8.65548074121795));
#44372=CARTESIAN_POINT('Ctrl Pts',(13.4704741473203,1.69147475074932,7.95472534478866));
#44373=CARTESIAN_POINT('Ctrl Pts',(13.4178734343653,0.870825559620414,7.49283066140558));
#44374=CARTESIAN_POINT('Ctrl Pts',(13.3652727214103,0.0426070147234524,
7.47883399491689));
#44375=CARTESIAN_POINT('Ctrl Pts',(13.3126720084553,-0.785611530173522,
7.46483732842821));
#44376=CARTESIAN_POINT('Ctrl Pts',(13.2600712955003,-1.62139942883856,7.89873867883393));
#44377=CARTESIAN_POINT('Ctrl Pts',(13.2074705825453,-2.08650844588355,8.58416954117274));
#44378=CARTESIAN_POINT('Ctrl Pts',(13.1758414891942,-2.36618101479215,8.99632282793861));
#44379=CARTESIAN_POINT('Ctrl Pts',(13.1442123958431,-2.51182788845302,9.49942118706689));
#44380=CARTESIAN_POINT('Ctrl Pts',(13.112583302492,-2.51415776047792,10.0012738589896));
#44381=CARTESIAN_POINT('Ctrl Pts',(13.387416697508,-2.52103810132661,10.001041928985));
#44382=CARTESIAN_POINT('Ctrl Pts',(13.4364120331305,-2.51698407552909,9.22908130753535));
#44383=CARTESIAN_POINT('Ctrl Pts',(13.4854073687531,-2.13598344491356,8.45365903697655));
#44384=CARTESIAN_POINT('Ctrl Pts',(13.5344027043756,-1.520510482961,7.98843310210574));
#44385=CARTESIAN_POINT('Ctrl Pts',(13.5871541408985,-0.857853875520787,
7.48754182214329));
#44386=CARTESIAN_POINT('Ctrl Pts',(13.6399055774215,0.0766035185270594,
7.34623074323072));
#44387=CARTESIAN_POINT('Ctrl Pts',(13.6926570139444,0.857735340163466,7.62878857970604));
#44388=CARTESIAN_POINT('Ctrl Pts',(13.7454084504673,1.63886716179986,7.91134641618136));
#44389=CARTESIAN_POINT('Ctrl Pts',(13.7981598869902,2.26667341102482,8.61777316804455));
#44390=CARTESIAN_POINT('Ctrl Pts',(13.8509113235132,2.45553701572534,9.42668378890823));
#44391=CARTESIAN_POINT('Ctrl Pts',(13.9036627600361,2.64440062042586,10.2355944097719));
#44392=CARTESIAN_POINT('Ctrl Pts',(13.956414196559,2.39432158060191,11.1469888996361));
#44393=CARTESIAN_POINT('Ctrl Pts',(14.009165633082,1.81907200865208,11.7462332435378));
#44394=CARTESIAN_POINT('Ctrl Pts',(14.0619170696049,1.24382243670226,12.3454775874394));
#44395=CARTESIAN_POINT('Ctrl Pts',(14.1146685061278,0.343402332626565,12.6325717853785));
#44396=CARTESIAN_POINT('Ctrl Pts',(14.1674199426507,-0.472547026325317,
12.4769038781125));
#44397=CARTESIAN_POINT('Ctrl Pts',(14.2201713791737,-1.28849638527722,12.3212359708466));
#44398=CARTESIAN_POINT('Ctrl Pts',(14.2729228156966,-2.01997499910531,11.7228059583755));
#44399=CARTESIAN_POINT('Ctrl Pts',(14.3256742522195,-2.33420061173484,10.9538663521032));
#44400=CARTESIAN_POINT('Ctrl Pts',(14.3462550673157,-2.45679479415481,10.6538668658346));
#44401=CARTESIAN_POINT('Ctrl Pts',(14.3668358824119,-2.51587694143337,10.327913315048));
#44402=CARTESIAN_POINT('Ctrl Pts',(14.387416697508,-2.5142305845587,10.0013871638039));
#44403=CARTESIAN_POINT('Origin',(17.,0.,10.));
#44404=CARTESIAN_POINT('',(15.387416697508,-2.51610609219152,9.99784272973747));
#44405=CARTESIAN_POINT('',(15.112583302492,-2.52097083132827,10.0010472664792));
#44406=CARTESIAN_POINT('',(17.,-2.5175,10.));
#44407=CARTESIAN_POINT('Ctrl Pts',(15.112583302492,-2.52097083132827,10.0010472664792));
#44408=CARTESIAN_POINT('Ctrl Pts',(15.1087542846364,-2.52129013078259,10.0613807422796));
#44409=CARTESIAN_POINT('Ctrl Pts',(15.1049252667809,-2.51930944209528,10.1216929066385));
#44410=CARTESIAN_POINT('Ctrl Pts',(15.1010962489253,-2.51496119606018,10.18183389453));
#44411=CARTESIAN_POINT('Ctrl Pts',(15.0484955359703,-2.45522764291969,11.0080141214861));
#44412=CARTESIAN_POINT('Ctrl Pts',(14.9958948230153,-1.94869838889795,11.8018906284176));
#44413=CARTESIAN_POINT('Ctrl Pts',(14.9432941100603,-1.22461077616291,12.2041828031708));
#44414=CARTESIAN_POINT('Ctrl Pts',(14.8906933971053,-0.500523163427894,
12.6064749779241));
#44415=CARTESIAN_POINT('Ctrl Pts',(14.8380926841503,0.441122808020406,12.6171828204993));
#44416=CARTESIAN_POINT('Ctrl Pts',(14.7854919711953,1.17417125864671,12.2314603375943));
#44417=CARTESIAN_POINT('Ctrl Pts',(14.7328912582403,1.90721970927303,11.8457378546893));
#44418=CARTESIAN_POINT('Ctrl Pts',(14.6802905452853,2.43167063907734,11.0635850463041));
#44419=CARTESIAN_POINT('Ctrl Pts',(14.6276898323303,2.51017598515645,10.2389767905723));
#44420=CARTESIAN_POINT('Ctrl Pts',(14.5750891193753,2.58868133123557,9.41436853484049));
#44421=CARTESIAN_POINT('Ctrl Pts',(14.5224884064203,2.22124109358949,8.5473048317621));
#44422=CARTESIAN_POINT('Ctrl Pts',(14.4698876934653,1.57414581282329,8.03018824684711));
#44423=CARTESIAN_POINT('Ctrl Pts',(14.4172869805103,0.927050532057081,7.51307166193211));
#44424=CARTESIAN_POINT('Ctrl Pts',(14.3646862675553,0.000300208170735533,
7.34590219518052));
#44425=CARTESIAN_POINT('Ctrl Pts',(14.3120855546003,-0.78669052599029,7.6043348733169));
#44426=CARTESIAN_POINT('Ctrl Pts',(14.2594848416453,-1.5736812601513,7.86276755145327));
#44427=CARTESIAN_POINT('Ctrl Pts',(14.2068841286903,-2.220912404587,8.54680237447761));
#44428=CARTESIAN_POINT('Ctrl Pts',(14.1542834157353,-2.43546988544923,9.34686921680396));
#44429=CARTESIAN_POINT('Ctrl Pts',(14.1403833779875,-2.49216792080863,9.55829143305017));
#44430=CARTESIAN_POINT('Ctrl Pts',(14.1264833402398,-2.51865189118754,9.77781628938327));
#44431=CARTESIAN_POINT('Ctrl Pts',(14.112583302492,-2.51674334939835,9.9977931730102));
#44432=CARTESIAN_POINT('Ctrl Pts',(14.387416697508,-2.5142305845587,10.0013871638039));
#44433=CARTESIAN_POINT('Ctrl Pts',(14.4195873189348,-2.51165710418384,9.49098224793788));
#44434=CARTESIAN_POINT('Ctrl Pts',(14.4517579403615,-2.3606998738868,8.97917824272694));
#44435=CARTESIAN_POINT('Ctrl Pts',(14.4839285617883,-2.07199020161617,8.56291610617037));
#44436=CARTESIAN_POINT('Ctrl Pts',(14.5366799983112,-1.598581567437,7.88035466658329));
#44437=CARTESIAN_POINT('Ctrl Pts',(14.5894314348342,-0.754791687647666,
7.45468098748261));
#44438=CARTESIAN_POINT('Ctrl Pts',(14.6421828713571,0.0755017760662482,
7.47955301676295));
#44439=CARTESIAN_POINT('Ctrl Pts',(14.69493430788,0.905795239780163,7.50442504604328));
#44440=CARTESIAN_POINT('Ctrl Pts',(14.747685744403,1.72259228741866,7.97984278370464));
#44441=CARTESIAN_POINT('Ctrl Pts',(14.8004371809259,2.15429550091668,8.68951749030059));
#44442=CARTESIAN_POINT('Ctrl Pts',(14.8531886174488,2.58599871441471,9.39919219689654));
#44443=CARTESIAN_POINT('Ctrl Pts',(14.9059400539717,2.63260809377225,10.3431238724271));
#44444=CARTESIAN_POINT('Ctrl Pts',(14.9586914904947,2.27291895285955,11.0918758845353));
#44445=CARTESIAN_POINT('Ctrl Pts',(15.0114429270176,1.91322981194686,11.8406278966435));
#44446=CARTESIAN_POINT('Ctrl Pts',(15.0641943635405,1.14724215076395,12.3942002453293));
#44447=CARTESIAN_POINT('Ctrl Pts',(15.1169458000635,0.32343793063549,12.5007481717526));
#44448=CARTESIAN_POINT('Ctrl Pts',(15.1696972365864,-0.500366289492972,
12.607296098176));
#44449=CARTESIAN_POINT('Ctrl Pts',(15.2224486731093,-1.38198706856698,12.2668196023368));
#44450=CARTESIAN_POINT('Ctrl Pts',(15.2752001096322,-1.92033578100497,11.6342166324236));
#44451=CARTESIAN_POINT('Ctrl Pts',(15.3126056389242,-2.30207360389097,11.1856440345767));
#44452=CARTESIAN_POINT('Ctrl Pts',(15.3500111682161,-2.51121114836557,10.5901876216538));
#44453=CARTESIAN_POINT('Ctrl Pts',(15.387416697508,-2.51610609219152,9.99784272973747));
#44454=CARTESIAN_POINT('Origin',(17.,0.,10.));
#44455=CARTESIAN_POINT('',(16.387416697508,-2.52148707396491,10.0004260768809));
#44456=CARTESIAN_POINT('',(16.112583302492,-2.51402132015258,10.00114820235));
#44457=CARTESIAN_POINT('',(17.,-2.5175,10.));
#44458=CARTESIAN_POINT('Ctrl Pts',(16.112583302492,-2.51402132015258,10.00114820235));
#44459=CARTESIAN_POINT('Ctrl Pts',(16.0910252290331,-2.51544798192459,10.3432525163187));
#44460=CARTESIAN_POINT('Ctrl Pts',(16.0694671555742,-2.45037630801831,10.6848371225185));
#44461=CARTESIAN_POINT('Ctrl Pts',(16.0479090821154,-2.31618714117941,10.9966797429082));
#44462=CARTESIAN_POINT('Ctrl Pts',(15.9953083691604,-1.9887717132641,11.7575614698192));
#44463=CARTESIAN_POINT('Ctrl Pts',(15.9427076562054,-1.24987381049529,12.3413779501632));
#44464=CARTESIAN_POINT('Ctrl Pts',(15.8901069432504,-0.433892660596432,
12.4839143588234));
#44465=CARTESIAN_POINT('Ctrl Pts',(15.8375062302954,0.38208848930245,12.6264507674836));
#44466=CARTESIAN_POINT('Ctrl Pts',(15.7849055173404,1.27515288633139,12.3277071044599));
#44467=CARTESIAN_POINT('Ctrl Pts',(15.7323048043854,1.8411309644993,11.7228842545134));
#44468=CARTESIAN_POINT('Ctrl Pts',(15.6797040914304,2.40710904266722,11.1180614045669));
#44469=CARTESIAN_POINT('Ctrl Pts',(15.6271033784754,2.6460008019741,10.2071593676976));
#44470=CARTESIAN_POINT('Ctrl Pts',(15.5745026655204,2.44969222623129,9.4024203989171));
#44471=CARTESIAN_POINT('Ctrl Pts',(15.5219019525654,2.25338365048847,8.59768143013662));
#44472=CARTESIAN_POINT('Ctrl Pts',(15.4693012396104,1.62187473969598,7.89910552944501));
#44473=CARTESIAN_POINT('Ctrl Pts',(15.4167005266554,0.840964237195962,7.62284360324235));
#44474=CARTESIAN_POINT('Ctrl Pts',(15.3640998137004,0.0600537346959255,
7.34658167703968));
#44475=CARTESIAN_POINT('Ctrl Pts',(15.3114991007454,-0.870258359511636,
7.492633725326));
#44476=CARTESIAN_POINT('Ctrl Pts',(15.2588983877904,-1.52894548048579,7.99490172295958));
#44477=CARTESIAN_POINT('Ctrl Pts',(15.2101266926909,-2.13968411168212,8.46060760910896));
#44478=CARTESIAN_POINT('Ctrl Pts',(15.1613549975914,-2.51690378953878,9.2325562337822));
#44479=CARTESIAN_POINT('Ctrl Pts',(15.112583302492,-2.52097083132827,10.0010472664792));
#44480=CARTESIAN_POINT('Ctrl Pts',(15.387416697508,-2.51610609219152,9.99784272973747));
#44481=CARTESIAN_POINT('Ctrl Pts',(15.402762604739,-2.51811428069402,9.75482866384464));
#44482=CARTESIAN_POINT('Ctrl Pts',(15.41810851197,-2.48574611148528,9.51233830240333));
#44483=CARTESIAN_POINT('Ctrl Pts',(15.433454419201,-2.41681664896408,9.28072898098979));
#44484=CARTESIAN_POINT('Ctrl Pts',(15.4862058557239,-2.17987215868322,8.48457374345623));
#44485=CARTESIAN_POINT('Ctrl Pts',(15.5389572922469,-1.51090653231955,7.81699271237621));
#44486=CARTESIAN_POINT('Ctrl Pts',(15.5917087287698,-0.714262078956731,
7.58169828266564));
#44487=CARTESIAN_POINT('Ctrl Pts',(15.6444601652927,0.0823823744060931,
7.34640385295507));
#44488=CARTESIAN_POINT('Ctrl Pts',(15.6972116018157,1.00670565476806,7.54339602461395));
#44489=CARTESIAN_POINT('Ctrl Pts',(15.7499630383386,1.63819186355563,8.08305427002273));
#44490=CARTESIAN_POINT('Ctrl Pts',(15.8027144748615,2.26967807234319,8.62271251543151));
#44491=CARTESIAN_POINT('Ctrl Pts',(15.8554659113844,2.60832720955635,9.50503683459018));
#44492=CARTESIAN_POINT('Ctrl Pts',(15.9082173479074,2.50007267397243,10.3286185301445));
#44493=CARTESIAN_POINT('Ctrl Pts',(15.9609687844303,2.3918181383885,11.1522002256988));
#44494=CARTESIAN_POINT('Ctrl Pts',(16.0137202209532,1.8366599300075,11.9170392976487));
#44495=CARTESIAN_POINT('Ctrl Pts',(16.0664716574762,1.08716428599743,12.2751763291555));
#44496=CARTESIAN_POINT('Ctrl Pts',(16.1192230939991,0.337668641987382,12.6333133606624));
#44497=CARTESIAN_POINT('Ctrl Pts',(16.171974530522,-0.606164437651727,12.5847483517261));
#44498=CARTESIAN_POINT('Ctrl Pts',(16.2247259670449,-1.31494317623276,12.1515756916216));
#44499=CARTESIAN_POINT('Ctrl Pts',(16.2774774035679,-2.02372191481378,11.718403031517));
#44500=CARTESIAN_POINT('Ctrl Pts',(16.3302288400908,-2.49744631233675,10.9006227202442));
#44501=CARTESIAN_POINT('Ctrl Pts',(16.3829802766137,-2.52059800533192,10.0702795063633));
#44502=CARTESIAN_POINT('Ctrl Pts',(16.3844590835785,-2.52124702812834,10.0470020866612));
#44503=CARTESIAN_POINT('Ctrl Pts',(16.3859378905433,-2.52154195635077,10.0237147940671));
#44504=CARTESIAN_POINT('Ctrl Pts',(16.387416697508,-2.52148707396491,10.0004260768809));
#44505=CARTESIAN_POINT('Origin',(17.,0.,10.));
#44506=CARTESIAN_POINT('',(17.387416697508,-2.5149367383853,10.0018020624789));
#44507=CARTESIAN_POINT('',(17.112583302492,-2.51701152631831,9.99777648906939));
#44508=CARTESIAN_POINT('',(17.,-2.5175,10.));
#44509=CARTESIAN_POINT('Ctrl Pts',(17.112583302492,-2.51701152631831,9.99777648906939));
#44510=CARTESIAN_POINT('Ctrl Pts',(17.0732961734298,-2.5115265699017,10.6193511875094));
#44511=CARTESIAN_POINT('Ctrl Pts',(17.0340090443676,-2.27855779157825,11.2446011064688));
#44512=CARTESIAN_POINT('Ctrl Pts',(16.9947219153054,-1.86114087724942,11.7012489582421));
#44513=CARTESIAN_POINT('Ctrl Pts',(16.9421212023504,-1.30227012702427,12.3126451876439));
#44514=CARTESIAN_POINT('Ctrl Pts',(16.8895204893954,-0.412758194743455,
12.6218058510013));
#44515=CARTESIAN_POINT('Ctrl Pts',(16.8369197764404,0.404833074321963,12.48881569523));
#44516=CARTESIAN_POINT('Ctrl Pts',(16.7843190634854,1.22242434338735,12.3558255394588));
#44517=CARTESIAN_POINT('Ctrl Pts',(16.7317183505304,1.96809494923736,11.780684564559));
#44518=CARTESIAN_POINT('Ctrl Pts',(16.6791176375754,2.30438057671027,11.0236813667196));
#44519=CARTESIAN_POINT('Ctrl Pts',(16.6265169246204,2.64066620418318,10.2666781688801));
#44520=CARTESIAN_POINT('Ctrl Pts',(16.5739162116654,2.56756685327896,9.32781274810094));
#44521=CARTESIAN_POINT('Ctrl Pts',(16.5213154987104,2.118164721684,8.63198260438628));
#44522=CARTESIAN_POINT('Ctrl Pts',(16.4687147857554,1.66876259008904,7.93615246067163));
#44523=CARTESIAN_POINT('Ctrl Pts',(16.4161140728004,0.843057677803332,7.48335759402149));
#44524=CARTESIAN_POINT('Ctrl Pts',(16.3635133598454,0.014735014871155,7.47851705097473));
#44525=CARTESIAN_POINT('Ctrl Pts',(16.3109126468904,-0.813587648061016,
7.47367650792798));
#44526=CARTESIAN_POINT('Ctrl Pts',(16.2583119339354,-1.64452806163966,7.91679028848459));
#44527=CARTESIAN_POINT('Ctrl Pts',(16.2057112209804,-2.10203179189809,8.60732066550189));
#44528=CARTESIAN_POINT('Ctrl Pts',(16.1746685814843,-2.37203047763264,9.01484148319913));
#44529=CARTESIAN_POINT('Ctrl Pts',(16.1436259419881,-2.51196699247083,9.50853364155139));
#44530=CARTESIAN_POINT('Ctrl Pts',(16.112583302492,-2.51402132015258,10.00114820235));
#44531=CARTESIAN_POINT('Ctrl Pts',(16.387416697508,-2.52148707396491,10.0004260768809));
#44532=CARTESIAN_POINT('Ctrl Pts',(16.4386893270662,-2.51958421287035,9.192968580655));
#44533=CARTESIAN_POINT('Ctrl Pts',(16.4899619566244,-2.09716665055828,8.38379855228885));
#44534=CARTESIAN_POINT('Ctrl Pts',(16.5412345861825,-1.43278785810852,7.925036755228));
#44535=CARTESIAN_POINT('Ctrl Pts',(16.5939860227054,-0.749247029422589,
7.45304333446249));
#44536=CARTESIAN_POINT('Ctrl Pts',(16.6467374592284,0.19041361641662,7.35196260942039));
#44537=CARTESIAN_POINT('Ctrl Pts',(16.6994888957513,0.958700529009151,7.66778071160203));
#44538=CARTESIAN_POINT('Ctrl Pts',(16.7522403322742,1.72698744160169,7.98359881378368));
#44539=CARTESIAN_POINT('Ctrl Pts',(16.8049917687972,2.32390062094753,8.71631574318908));
#44540=CARTESIAN_POINT('Ctrl Pts',(16.8577432053201,2.47787763070436,9.53258587874038));
#44541=CARTESIAN_POINT('Ctrl Pts',(16.910494641843,2.63185464046118,10.3488560142917));
#44542=CARTESIAN_POINT('Ctrl Pts',(16.9632460783659,2.342895480629,11.2486793559889));
#44543=CARTESIAN_POINT('Ctrl Pts',(17.0159975148889,1.74246056482014,11.8226861204126));
#44544=CARTESIAN_POINT('Ctrl Pts',(17.0687489514118,1.14202564901128,12.3966928848363));
#44545=CARTESIAN_POINT('Ctrl Pts',(17.1215003879347,0.230114977225762,12.6448830719865));
#44546=CARTESIAN_POINT('Ctrl Pts',(17.1742518244576,-0.578402601388186,
12.4543438928164));
#44547=CARTESIAN_POINT('Ctrl Pts',(17.2270032609806,-1.38692018000214,12.2638047136463));
#44548=CARTESIAN_POINT('Ctrl Pts',(17.2797546975035,-2.09204466544451,11.6345361681559));
#44549=CARTESIAN_POINT('Ctrl Pts',(17.3325061340264,-2.37298347042277,10.8528205922691));
#44550=CARTESIAN_POINT('Ctrl Pts',(17.350809655187,-2.47046269943862,10.5815834748014));
#44551=CARTESIAN_POINT('Ctrl Pts',(17.3691131763475,-2.51687300377292,10.2919928242661));
#44552=CARTESIAN_POINT('Ctrl Pts',(17.387416697508,-2.5149367383853,10.0018020624789));
#44553=CARTESIAN_POINT('Origin',(17.,0.,10.));
#44554=CARTESIAN_POINT('',(18.387416697508,-2.51518334819126,9.99809619657404));
#44555=CARTESIAN_POINT('',(18.112583302492,-2.5208033701771,10.0011896703713));
#44556=CARTESIAN_POINT('',(17.,-2.5175,10.));
#44557=CARTESIAN_POINT('Ctrl Pts',(18.112583302492,-2.5208033701771,10.0011896703713));
#44558=CARTESIAN_POINT('Ctrl Pts',(18.1081678307815,-2.52121299156672,10.0707760983448));
#44559=CARTESIAN_POINT('Ctrl Pts',(18.103752359071,-2.51857806098439,10.1403310528238));
#44560=CARTESIAN_POINT('Ctrl Pts',(18.0993368873605,-2.5127975112366,10.2096235922112));
#44561=CARTESIAN_POINT('Ctrl Pts',(18.0467361744055,-2.44393487142343,11.03509303539));
#44562=CARTESIAN_POINT('Ctrl Pts',(17.9941354614505,-1.92866092038828,11.8233217768237));
#44563=CARTESIAN_POINT('Ctrl Pts',(17.9415347484955,-1.20017054290006,12.2175851845743));
#44564=CARTESIAN_POINT('Ctrl Pts',(17.8889340355405,-0.47168016541185,12.6118485923249));
#44565=CARTESIAN_POINT('Ctrl Pts',(17.8363333225855,0.470026638529419,12.6121466663925));
#44566=CARTESIAN_POINT('Ctrl Pts',(17.7837326096305,1.19876645873966,12.2183445089276));
#44567=CARTESIAN_POINT('Ctrl Pts',(17.7311318966755,1.92750627894991,11.8245423514627));
#44568=CARTESIAN_POINT('Ctrl Pts',(17.6785311837205,2.44327911542912,11.0366399624654));
#44569=CARTESIAN_POINT('Ctrl Pts',(17.6259304707655,2.51266430538601,10.2112142782281));
#44570=CARTESIAN_POINT('Ctrl Pts',(17.5733297578105,2.58204949534291,9.38578859399074));
#44571=CARTESIAN_POINT('Ctrl Pts',(17.5207290448555,2.20504703877749,8.52283961451336));
#44572=CARTESIAN_POINT('Ctrl Pts',(17.4681283319005,1.55227500058467,8.01290772598547));
#44573=CARTESIAN_POINT('Ctrl Pts',(17.4155276189455,0.899502962391848,7.50297583745757));
#44574=CARTESIAN_POINT('Ctrl Pts',(17.3629269059905,-0.0290386574283893,
7.34606103987917));
#44575=CARTESIAN_POINT('Ctrl Pts',(17.3103261930355,-0.813124548432665,
7.61317745703109));
#44576=CARTESIAN_POINT('Ctrl Pts',(17.2577254800805,-1.59721043943693,7.880293874183));
#44577=CARTESIAN_POINT('Ctrl Pts',(17.2051247671255,-2.23684060162524,8.57144150606521));
#44578=CARTESIAN_POINT('Ctrl Pts',(17.1525240541704,-2.44254089863465,9.3738312197295));
#44579=CARTESIAN_POINT('Ctrl Pts',(17.1392104702776,-2.49460498687914,9.57692129527171));
#44580=CARTESIAN_POINT('Ctrl Pts',(17.1258968863848,-2.51887026298714,9.78713786286086));
#44581=CARTESIAN_POINT('Ctrl Pts',(17.112583302492,-2.51701152631831,9.99777648906939));
#44582=CARTESIAN_POINT('Ctrl Pts',(17.387416697508,-2.5149367383853,10.0018020624789));
#44583=CARTESIAN_POINT('Ctrl Pts',(17.4218646128704,-2.51129261408774,9.45565213245618));
#44584=CARTESIAN_POINT('Ctrl Pts',(17.4563125282328,-2.33640176855005,8.9073765690155));
#44585=CARTESIAN_POINT('Ctrl Pts',(17.4907604435952,-2.00841223852946,8.47532502033285));
#44586=CARTESIAN_POINT('Ctrl Pts',(17.5435118801181,-1.50614907714372,7.81370763056639));
#44587=CARTESIAN_POINT('Ctrl Pts',(17.5962633166411,-0.644869629858092,
7.42463545731654));
#44588=CARTESIAN_POINT('Ctrl Pts',(17.649014753164,0.1835916570973,7.48511479050391));
#44589=CARTESIAN_POINT('Ctrl Pts',(17.7017661896869,1.01205294405269,7.54559412369128));
#44590=CARTESIAN_POINT('Ctrl Pts',(17.7545176262099,1.80769607067784,8.05562496331587));
#44591=CARTESIAN_POINT('Ctrl Pts',(17.8072690627328,2.20854748135092,8.78317152559761));
#44592=CARTESIAN_POINT('Ctrl Pts',(17.8600204992557,2.609398892024,9.51071808787935));
#44593=CARTESIAN_POINT('Ctrl Pts',(17.9127719357786,2.615458586745,10.4557803728183));
#44594=CARTESIAN_POINT('Ctrl Pts',(17.9655233723016,2.22396974003433,11.1884073833958));
#44595=CARTESIAN_POINT('Ctrl Pts',(18.0182748088245,1.83248089332367,11.9210343939733));
#44596=CARTESIAN_POINT('Ctrl Pts',(18.0710262453474,1.04344350518134,12.4412261301894));
#44597=CARTESIAN_POINT('Ctrl Pts',(18.1237776818704,0.215825886080791,12.51232416308));
#44598=CARTESIAN_POINT('Ctrl Pts',(18.1765291183933,-0.611791733019759,
12.5834221959705));
#44599=CARTESIAN_POINT('Ctrl Pts',(18.2292805549162,-1.47798958307853,12.2054265255356));
#44600=CARTESIAN_POINT('Ctrl Pts',(18.2820319914391,-1.98869561701118,11.5503042463912));
#44601=CARTESIAN_POINT('Ctrl Pts',(18.3171602267954,-2.32878496699634,11.1140452338251));
#44602=CARTESIAN_POINT('Ctrl Pts',(18.3522884621517,-2.51123167916713,10.5548945888113));
#44603=CARTESIAN_POINT('Ctrl Pts',(18.387416697508,-2.51518334819126,9.99809619657404));
#44604=CARTESIAN_POINT('Origin',(17.,0.,10.));
#44605=CARTESIAN_POINT('',(19.387416697508,-2.52155059213328,9.99976874863484));
#44606=CARTESIAN_POINT('',(19.112583302492,-2.51389966012859,10.0010175250377));
#44607=CARTESIAN_POINT('',(17.,-2.5175,10.));
#44608=CARTESIAN_POINT('Ctrl Pts',(19.112583302492,-2.51389966012859,10.0010175250377));
#44609=CARTESIAN_POINT('Ctrl Pts',(19.0904387751782,-2.51519458398436,10.3524708738624));
#44610=CARTESIAN_POINT('Ctrl Pts',(19.0682942478644,-2.4464002454655,10.7034398319222));
#44611=CARTESIAN_POINT('Ctrl Pts',(19.0461497205505,-2.30502815708954,11.0222223720467));
#44612=CARTESIAN_POINT('Ctrl Pts',(18.9935490075955,-1.96922181834357,11.7794383040252));
#44613=CARTESIAN_POINT('Ctrl Pts',(18.9409482946405,-1.22391545525877,12.355051210919));
#44614=CARTESIAN_POINT('Ctrl Pts',(18.8883475816855,-0.406408539519951,
12.4885589167013));
#44615=CARTESIAN_POINT('Ctrl Pts',(18.8357468687305,0.411098376218855,12.6220666224836));
#44616=CARTESIAN_POINT('Ctrl Pts',(18.7831461557755,1.30080584461167,12.3134691271544));
#44617=CARTESIAN_POINT('Ctrl Pts',(18.7305454428205,1.86006352761385,11.7024268137365));
#44618=CARTESIAN_POINT('Ctrl Pts',(18.6779447298655,2.41932121061604,11.0913845003187));
#44619=CARTESIAN_POINT('Ctrl Pts',(18.6253440169105,2.64812910822757,10.1778973688121));
#44620=CARTESIAN_POINT('Ctrl Pts',(18.5727433039555,2.44293680574081,9.37537759722749));
#44621=CARTESIAN_POINT('Ctrl Pts',(18.5201425910005,2.23774450325404,8.57285782564289));
#44622=CARTESIAN_POINT('Ctrl Pts',(18.4675418780455,1.59855200066899,7.8813054139802));
#44623=CARTESIAN_POINT('Ctrl Pts',(18.4149411650905,0.814635364990448,7.61369268429331));
#44624=CARTESIAN_POINT('Ctrl Pts',(18.3623404521355,0.0307187293118991,
7.34607995460641));
#44625=CARTESIAN_POINT('Ctrl Pts',(18.3097397391805,-0.897922039460136,
7.50240690689532));
#44626=CARTESIAN_POINT('Ctrl Pts',(18.2571390262255,-1.55101675955056,8.01192545550181));
#44627=CARTESIAN_POINT('Ctrl Pts',(18.208953784981,-2.14928862461043,8.47867339110784));
#44628=CARTESIAN_POINT('Ctrl Pts',(18.1607685437365,-2.51633324631003,9.24180561378778));
#44629=CARTESIAN_POINT('Ctrl Pts',(18.112583302492,-2.5208033701771,10.0011896703713));
#44630=CARTESIAN_POINT('Ctrl Pts',(18.387416697508,-2.51518334819126,9.99809619657404));
#44631=CARTESIAN_POINT('Ctrl Pts',(18.4050398986747,-2.51716582916276,9.71876050048428));
#44632=CARTESIAN_POINT('Ctrl Pts',(18.4226630998413,-2.474223826934,9.44001683058457));
#44633=CARTESIAN_POINT('Ctrl Pts',(18.4402863010079,-2.3837243979264,9.17767919384928));
#44634=CARTESIAN_POINT('Ctrl Pts',(18.4930377375309,-2.11283292710244,8.39242530830563));
#44635=CARTESIAN_POINT('Ctrl Pts',(18.5457891740538,-1.41583576764798,7.75416642507215));
#44636=CARTESIAN_POINT('Ctrl Pts',(18.5985406105767,-0.609828023666041,
7.55327498581276));
#44637=CARTESIAN_POINT('Ctrl Pts',(18.6512920470996,0.196179720315914,7.35238354655336));
#44638=CARTESIAN_POINT('Ctrl Pts',(18.7040434836226,1.11119804882536,7.58885955126807));
#44639=CARTESIAN_POINT('Ctrl Pts',(18.7567949201455,1.71894430102338,8.15511951512376));
#44640=CARTESIAN_POINT('Ctrl Pts',(18.8095463566684,2.32669055322138,8.72137947897945));
#44641=CARTESIAN_POINT('Ctrl Pts',(18.8622977931914,2.62716472910797,9.61742340197613));
#44642=CARTESIAN_POINT('Ctrl Pts',(18.9150492297143,2.48366772052954,10.4356009268786));
#44643=CARTESIAN_POINT('Ctrl Pts',(18.9678006662372,2.34017071195111,11.2537784517812));
#44644=CARTESIAN_POINT('Ctrl Pts',(19.0205521027601,1.75270251890765,11.9940895785895));
#44645=CARTESIAN_POINT('Ctrl Pts',(19.0733035392831,0.988528632087992,12.319733747015));
#44646=CARTESIAN_POINT('Ctrl Pts',(19.126054975806,0.224354745268327,12.6453779154405));
#44647=CARTESIAN_POINT('Ctrl Pts',(19.1788064123289,-0.716524835327532,
12.556355125483));
#44648=CARTESIAN_POINT('Ctrl Pts',(19.2315578488519,-1.40606201149648,12.0931658160128));
#44649=CARTESIAN_POINT('Ctrl Pts',(19.2835107984039,-2.08516181406211,11.6369877019343));
#44650=CARTESIAN_POINT('Ctrl Pts',(19.335463747956,-2.52047065422532,10.8178846922386));
#44651=CARTESIAN_POINT('Ctrl Pts',(19.387416697508,-2.52155059213328,9.99976874863484));
#44652=CARTESIAN_POINT('Origin',(17.,0.,10.));
#44653=CARTESIAN_POINT('',(20.387416697508,-2.5158164891674,10.0020963764446));
#44654=CARTESIAN_POINT('',(20.112583302492,-2.51728339305687,9.99777041742395));
#44655=CARTESIAN_POINT('',(17.,-2.5175,10.));
#44656=CARTESIAN_POINT('Ctrl Pts',(20.112583302492,-2.51728339305687,9.99777041742395));
#44657=CARTESIAN_POINT('Ctrl Pts',(20.0727097195748,-2.51164716853644,10.6284495053142));
#44658=CARTESIAN_POINT('Ctrl Pts',(20.0328361366577,-2.27096645283767,11.2629653655237));
#44659=CARTESIAN_POINT('Ctrl Pts',(19.9929625537406,-1.84222126852405,11.7217183801906));
#44660=CARTESIAN_POINT('Ctrl Pts',(19.9403618407856,-1.27662618724459,12.3268994017176));
#44661=CARTESIAN_POINT('Ctrl Pts',(19.8877611278306,-0.383751089025701,
12.6262083598496));
#44662=CARTESIAN_POINT('Ctrl Pts',(19.8351604148756,0.432320130131445,12.4841885371227));
#44663=CARTESIAN_POINT('Ctrl Pts',(19.7825597019206,1.2483913492886,12.3421687143957));
#44664=CARTESIAN_POINT('Ctrl Pts',(19.7299589889656,1.98765868938402,11.7588201108097));
#44665=CARTESIAN_POINT('Ctrl Pts',(19.6773582760106,2.31555572834135,10.9981458069009));
#44666=CARTESIAN_POINT('Ctrl Pts',(19.6247575630556,2.64345276729868,10.2374715029922));
#44667=CARTESIAN_POINT('Ctrl Pts',(19.5721568501006,2.55997950511793,9.29947149876068));
#44668=CARTESIAN_POINT('Ctrl Pts',(19.5195561371456,2.10291300721531,8.60865163708974));
#44669=CARTESIAN_POINT('Ctrl Pts',(19.4669554241906,1.64584650931268,7.91783177541879));
#44670=CARTESIAN_POINT('Ctrl Pts',(19.4143547112356,0.815186775688189,7.47419205630841));
#44671=CARTESIAN_POINT('Ctrl Pts',(19.3617539982806,-0.0131387855763111,
7.47850822821053));
#44672=CARTESIAN_POINT('Ctrl Pts',(19.3091532853256,-0.841464346840806,
7.48282440011265));
#44673=CARTESIAN_POINT('Ctrl Pts',(19.2565525723705,-1.66745573574531,7.93509646302726));
#44674=CARTESIAN_POINT('Ctrl Pts',(19.2039518594155,-2.11729827299398,8.63064197301616));
#44675=CARTESIAN_POINT('Ctrl Pts',(19.1734956737744,-2.37776029059948,9.03336775341074));
#44676=CARTESIAN_POINT('Ctrl Pts',(19.1430394881332,-2.51211870356159,9.51765076428747));
#44677=CARTESIAN_POINT('Ctrl Pts',(19.112583302492,-2.51389966012859,10.0010175250377));
#44678=CARTESIAN_POINT('Ctrl Pts',(19.387416697508,-2.52155059213328,9.99976874863484));
#44679=CARTESIAN_POINT('Ctrl Pts',(19.3882151844789,-2.52156719015815,9.98719477685344));
#44680=CARTESIAN_POINT('Ctrl Pts',(19.3890136714498,-2.52148121496597,9.97462103823604));
#44681=CARTESIAN_POINT('Ctrl Pts',(19.3898121584206,-2.52129197516155,9.96204885398458));
#44682=CARTESIAN_POINT('Ctrl Pts',(19.4425635949436,-2.50878999091566,9.1314770304097));
#44683=CARTESIAN_POINT('Ctrl Pts',(19.4953150314665,-2.0455912506818,8.30768921224301));
#44684=CARTESIAN_POINT('Ctrl Pts',(19.5480664679894,-1.34242552683065,7.8654632309535));
#44685=CARTESIAN_POINT('Ctrl Pts',(19.6008179045124,-0.639259802979503,
7.423237249664));
#44686=CARTESIAN_POINT('Ctrl Pts',(19.6535693410353,0.30387290448894,7.36257310525166));
#44687=CARTESIAN_POINT('Ctrl Pts',(19.7063207775582,1.0578994494348,7.71106962351769));
#44688=CARTESIAN_POINT('Ctrl Pts',(19.7590722140811,1.81192599438068,8.05956614178372));
#44689=CARTESIAN_POINT('Ctrl Pts',(19.811823650604,2.37684637680396,8.81722332272812));
#44690=CARTESIAN_POINT('Ctrl Pts',(19.864575087127,2.49565311102915,9.63934911214806));
#44691=CARTESIAN_POINT('Ctrl Pts',(19.9173265236499,2.61445984525433,10.461474901568));
#44692=CARTESIAN_POINT('Ctrl Pts',(19.9700779601728,2.2871529312814,11.3480692994635));
#44693=CARTESIAN_POINT('Ctrl Pts',(20.0228293966958,1.66263888695187,11.8957809591547));
#44694=CARTESIAN_POINT('Ctrl Pts',(20.0755808332187,1.03812484262234,12.443492618846));
#44695=CARTESIAN_POINT('Ctrl Pts',(20.1283322697416,0.116403667936205,12.6523215403331));
#44696=CARTESIAN_POINT('Ctrl Pts',(20.1810837062646,-0.683192552496604,
12.4272621304076));
#44697=CARTESIAN_POINT('Ctrl Pts',(20.2338351427875,-1.48278877292941,12.2022027204822));
#44698=CARTESIAN_POINT('Ctrl Pts',(20.2865865793104,-2.16026003910891,11.5432549791442));
#44699=CARTESIAN_POINT('Ctrl Pts',(20.3393380158334,-2.40739444692378,10.7502036326345));
#44700=CARTESIAN_POINT('Ctrl Pts',(20.3553642430582,-2.48247547666995,10.5092695099277));
#44701=CARTESIAN_POINT('Ctrl Pts',(20.3713904702831,-2.51783711775732,10.2559578436506));
#44702=CARTESIAN_POINT('Ctrl Pts',(20.387416697508,-2.5158164891674,10.0020963764446));
#44703=CARTESIAN_POINT('Origin',(17.,0.,10.));
#44704=CARTESIAN_POINT('',(21.387416697508,-2.51442093719447,9.99847790324227));
#44705=CARTESIAN_POINT('',(21.112583302492,-2.5206186296165,10.0013249946411));
#44706=CARTESIAN_POINT('',(17.,-2.5175,10.));
#44707=CARTESIAN_POINT('Ctrl Pts',(21.112583302492,-2.5206186296165,10.0013249946411));
#44708=CARTESIAN_POINT('Ctrl Pts',(21.1075813769266,-2.52112526980945,10.0801690222653));
#44709=CARTESIAN_POINT('Ctrl Pts',(21.1025794513611,-2.51774238317523,10.1589690246946));
#44710=CARTESIAN_POINT('Ctrl Pts',(21.0975775257956,-2.51032676658054,10.2373876742263));
#44711=CARTESIAN_POINT('Ctrl Pts',(21.0449768128406,-2.43234345499833,11.0620454625851));
#44712=CARTESIAN_POINT('Ctrl Pts',(20.9923760998856,-1.90838777260282,11.8445301182286));
#44713=CARTESIAN_POINT('Ctrl Pts',(20.9397753869306,-1.17558365071925,12.2307165806189));
#44714=CARTESIAN_POINT('Ctrl Pts',(20.8871746739756,-0.442779528835683,
12.6169030430092));
#44715=CARTESIAN_POINT('Ctrl Pts',(20.8345739610206,0.498873032535946,12.6067913121462));
#44716=CARTESIAN_POINT('Ctrl Pts',(20.7819732480656,1.22321517149131,12.2049576021148));
#44717=CARTESIAN_POINT('Ctrl Pts',(20.7293725351106,1.94755731044668,11.8031238920834));
#44718=CARTESIAN_POINT('Ctrl Pts',(20.6767718221556,2.45458902698578,11.0095682028835));
#44719=CARTESIAN_POINT('Ctrl Pts',(20.6241711092006,2.51484558206126,10.1834259558372));
#44720=CARTESIAN_POINT('Ctrl Pts',(20.5715703962456,2.57510213713674,9.35728370879087));
#44721=CARTESIAN_POINT('Ctrl Pts',(20.5189696832906,2.18858353074863,8.49855490389815));
#44722=CARTESIAN_POINT('Ctrl Pts',(20.4663689703356,1.53021450282693,7.99587002461758));
#44723=CARTESIAN_POINT('Ctrl Pts',(20.4137682573806,0.871845474905217,7.49318514533701));
#44724=CARTESIAN_POINT('Ctrl Pts',(20.3611675444256,-0.0583739745500803,
7.34654419166858));
#44725=CARTESIAN_POINT('Ctrl Pts',(20.3085668314706,-0.839459208357427,
7.6223117066376));
#44726=CARTESIAN_POINT('Ctrl Pts',(20.2559661185156,-1.62054444216476,7.89807922160661));
#44727=CARTESIAN_POINT('Ctrl Pts',(20.2033654055606,-2.25249546032415,8.59625520521304));
#44728=CARTESIAN_POINT('Ctrl Pts',(20.1507646926056,-2.44931343723384,9.40086973947727));
#44729=CARTESIAN_POINT('Ctrl Pts',(20.1380375625677,-2.49693499681351,9.59555215408064));
#44730=CARTESIAN_POINT('Ctrl Pts',(20.1253104325298,-2.51908240275568,9.79646583989391));
#44731=CARTESIAN_POINT('Ctrl Pts',(20.112583302492,-2.51728339305687,9.99777041742395));
#44732=CARTESIAN_POINT('Ctrl Pts',(20.387416697508,-2.5158164891674,10.0020963764446));
#44733=CARTESIAN_POINT('Ctrl Pts',(20.424141906806,-2.51118607885081,9.42035524766764));
#44734=CARTESIAN_POINT('Ctrl Pts',(20.4608671161041,-2.31025054570517,8.8357269550081));
#44735=CARTESIAN_POINT('Ctrl Pts',(20.4975923254021,-1.94113406353733,8.39054292978191));
#44736=CARTESIAN_POINT('Ctrl Pts',(20.550343761925,-1.41094172288576,7.75108852512045));
#44737=CARTESIAN_POINT('Ctrl Pts',(20.603095198448,-0.533759492132356,7.39933466747897));
#44738=CARTESIAN_POINT('Ctrl Pts',(20.6558466349709,0.291343296794607,7.49530988006332));
#44739=CARTESIAN_POINT('Ctrl Pts',(20.7085980714939,1.11644608572156,7.59128509264767));
#44740=CARTESIAN_POINT('Ctrl Pts',(20.7613495080168,1.88946943282209,8.13498937545785));
#44741=CARTESIAN_POINT('Ctrl Pts',(20.8141009445397,2.25873052935675,8.87906739308414));
#44742=CARTESIAN_POINT('Ctrl Pts',(20.8668523810626,2.62799162589142,9.62314541071043));
#44743=CARTESIAN_POINT('Ctrl Pts',(20.9196038175855,2.59349047186024,10.5675971631528));
#44744=CARTESIAN_POINT('Ctrl Pts',(20.9723552541085,2.17092318148099,11.2827494118573));
#44745=CARTESIAN_POINT('Ctrl Pts',(21.0251066906314,1.74835589110173,11.9979016605619));
#44746=CARTESIAN_POINT('Ctrl Pts',(21.0778581271544,0.937722464374398,12.4837544055285));
#44747=CARTESIAN_POINT('Ctrl Pts',(21.1306095636773,0.107816213237538,12.5192715569468));
#44748=CARTESIAN_POINT('Ctrl Pts',(21.1833610002002,-0.722090037899322,
12.5547887083651));
#44749=CARTESIAN_POINT('Ctrl Pts',(21.2361124367231,-1.57126911344571,12.1399702662351));
#44750=CARTESIAN_POINT('Ctrl Pts',(21.288863873246,-2.05339156615543,11.4635356468258));
#44751=CARTESIAN_POINT('Ctrl Pts',(21.3217148146667,-2.35363318032772,11.0422861885773));
#44752=CARTESIAN_POINT('Ctrl Pts',(21.3545657560874,-2.51152392557026,10.5195774789631));
#44753=CARTESIAN_POINT('Ctrl Pts',(21.387416697508,-2.51442093719447,9.99847790324227));
#44754=CARTESIAN_POINT('Origin',(17.,0.,10.));
#44755=CARTESIAN_POINT('',(22.387416697508,-2.52120696757832,9.99913427807354));
#44756=CARTESIAN_POINT('',(22.112583302492,-2.51379319101573,10.0008824115804));
#44757=CARTESIAN_POINT('',(17.,-2.5175,10.));
#44758=CARTESIAN_POINT('Ctrl Pts',(22.112583302492,-2.51379319101573,10.0008824115804));
#44759=CARTESIAN_POINT('Ctrl Pts',(22.0898523213232,-2.51494301618215,10.3616815724226));
#44760=CARTESIAN_POINT('Ctrl Pts',(22.0671213401545,-2.44231188243548,10.7220393548632));
#44761=CARTESIAN_POINT('Ctrl Pts',(22.0443903589857,-2.29358750221295,11.0476400873122));
#44762=CARTESIAN_POINT('Ctrl Pts',(21.9917896460307,-1.94943128759939,11.8010976938417));
#44763=CARTESIAN_POINT('Ctrl Pts',(21.9391889330757,-1.19780753951549,12.3684366881852));
#44764=CARTESIAN_POINT('Ctrl Pts',(21.8865882201207,-0.378874755990178,
12.4928993766318));
#44765=CARTESIAN_POINT('Ctrl Pts',(21.8339875071657,0.440058027535147,12.6173620650784));
#44766=CARTESIAN_POINT('Ctrl Pts',(21.7813867942107,1.32629984650189,12.2989484476281));
#44767=CARTESIAN_POINT('Ctrl Pts',(21.7287860812557,1.8787687939542,11.6817613391465));
#44768=CARTESIAN_POINT('Ctrl Pts',(21.6761853683007,2.4312377414065,11.064574230665));
#44769=CARTESIAN_POINT('Ctrl Pts',(21.6235846553457,2.64993381734437,10.1486136311522));
#44770=CARTESIAN_POINT('Ctrl Pts',(21.5709839423907,2.43588286227969,9.34841112338628));
#44771=CARTESIAN_POINT('Ctrl Pts',(21.5183832294356,2.221831907215,8.54820861562035));
#44772=CARTESIAN_POINT('Ctrl Pts',(21.4657825164807,1.57503392114776,7.86376419960125));
#44773=CARTESIAN_POINT('Ctrl Pts',(21.4131818035257,0.788206945650621,7.60483336828132));
#44774=CARTESIAN_POINT('Ctrl Pts',(21.3605810905707,0.00137997015348126,
7.3459025369614));
#44775=CARTESIAN_POINT('Ctrl Pts',(21.3079803776156,-0.925475994773556,
7.51248529034064));
#44776=CARTESIAN_POINT('Ctrl Pts',(21.2553796646606,-1.57289850685262,8.0291921275672));
#44777=CARTESIAN_POINT('Ctrl Pts',(21.2077808772711,-2.15875608885959,8.49676409582006));
#44778=CARTESIAN_POINT('Ctrl Pts',(21.1601820898816,-2.51579739457182,9.25103791845196));
#44779=CARTESIAN_POINT('Ctrl Pts',(21.112583302492,-2.5206186296165,10.0013249946411));
#44780=CARTESIAN_POINT('Ctrl Pts',(21.387416697508,-2.51442093719447,9.99847790324227));
#44781=CARTESIAN_POINT('Ctrl Pts',(21.4073171926103,-2.51617589346499,9.68280538044796));
#44782=CARTESIAN_POINT('Ctrl Pts',(21.4272176877126,-2.46105259485335,9.36772336364112));
#44783=CARTESIAN_POINT('Ctrl Pts',(21.4471181828148,-2.34624047609594,9.07614441500762));
#44784=CARTESIAN_POINT('Ctrl Pts',(21.4998696193378,-2.0419011034537,8.30323859928707));
#44785=CARTESIAN_POINT('Ctrl Pts',(21.5526210558607,-1.31815652829618,7.69547776453441));
#44786=CARTESIAN_POINT('Ctrl Pts',(21.6053724923836,-0.504270447552835,
7.52935942940694));
#44787=CARTESIAN_POINT('Ctrl Pts',(21.6581239289065,0.309615633190516,7.36324109427946));
#44788=CARTESIAN_POINT('Ctrl Pts',(21.7108753654295,1.2136432195197,7.63876525877716));
#44789=CARTESIAN_POINT('Ctrl Pts',(21.7636268019524,1.79652982974861,8.23058368824306));
#44790=CARTESIAN_POINT('Ctrl Pts',(21.8163782384753,2.37941643997752,8.82240211770896));
#44791=CARTESIAN_POINT('Ctrl Pts',(21.8691296749983,2.64116207410616,9.73051481214307));
#44792=CARTESIAN_POINT('Ctrl Pts',(21.9218811115212,2.46268696512556,10.5417807913922));
#44793=CARTESIAN_POINT('Ctrl Pts',(21.9746325480441,2.28421185614497,11.3530467706413));
#44794=CARTESIAN_POINT('Ctrl Pts',(22.0273839845671,1.66551600405516,12.0674660347054));
#44795=CARTESIAN_POINT('Ctrl Pts',(22.08013542109,0.888071755549521,12.360017387483));
#44796=CARTESIAN_POINT('Ctrl Pts',(22.1328868576129,0.11062750704388,12.6525687402605));
#44797=CARTESIAN_POINT('Ctrl Pts',(22.1856382941358,-0.82556513787759,12.5232521817515));
#44798=CARTESIAN_POINT('Ctrl Pts',(22.2383897306588,-1.49459037849252,12.0308995825432));
#44799=CARTESIAN_POINT('Ctrl Pts',(22.2880653862752,-2.12460672765935,11.5672546133773));
#44800=CARTESIAN_POINT('Ctrl Pts',(22.3377410418916,-2.51770286914662,10.7816745100176));
#44801=CARTESIAN_POINT('Ctrl Pts',(22.387416697508,-2.52120696757832,9.99913427807354));
#44802=CARTESIAN_POINT('Origin',(17.,0.,10.));
#44803=CARTESIAN_POINT('',(23.387416697508,-2.51682157436921,10.00224693272));
#44804=CARTESIAN_POINT('',(23.112583302492,-2.51755781857958,9.99777508489969));
#44805=CARTESIAN_POINT('',(17.,-2.5175,10.));
#44806=CARTESIAN_POINT('Ctrl Pts',(23.112583302492,-2.51755781857958,9.99777508489969));
#44807=CARTESIAN_POINT('Ctrl Pts',(23.0721232657199,-2.51179213810653,10.6375515055505));
#44808=CARTESIAN_POINT('Ctrl Pts',(23.0316632289478,-2.26324677579117,11.2813147064433));
#44809=CARTESIAN_POINT('Ctrl Pts',(22.9912031921757,-1.82307654140638,11.7419774141668));
#44810=CARTESIAN_POINT('Ctrl Pts',(22.9386024792207,-1.25082624216336,12.3408692786139));
#44811=CARTESIAN_POINT('Ctrl Pts',(22.8860017662657,-0.354697089633438,
12.6302899500812));
#44812=CARTESIAN_POINT('Ctrl Pts',(22.8334010533107,0.459754356125098,12.4792578134635));
#44813=CARTESIAN_POINT('Ctrl Pts',(22.7808003403557,1.27420580188363,12.3282256768458));
#44814=CARTESIAN_POINT('Ctrl Pts',(22.7281996274007,2.00697954087078,11.736740732143));
#44815=CARTESIAN_POINT('Ctrl Pts',(22.6755989144457,2.3264479232838,10.9724882761411));
#44816=CARTESIAN_POINT('Ctrl Pts',(22.6229982014907,2.64591630569681,10.2082358201392));
#44817=CARTESIAN_POINT('Ctrl Pts',(22.5703974885357,2.5520793315357,9.27121585283808));
#44818=CARTESIAN_POINT('Ctrl Pts',(22.5177967755807,2.08740431987843,8.5854906898792));
#44819=CARTESIAN_POINT('Ctrl Pts',(22.4651960626257,1.62272930822116,7.8997655269203));
#44820=CARTESIAN_POINT('Ctrl Pts',(22.4125953496707,0.787216259067707,7.46533516830362));
#44821=CARTESIAN_POINT('Ctrl Pts',(22.3599946367157,-0.0410109803468926,
7.47880752793945));
#44822=CARTESIAN_POINT('Ctrl Pts',(22.3073939237607,-0.869238219761481,
7.49227988757529));
#44823=CARTESIAN_POINT('Ctrl Pts',(22.2547932108057,-1.69017964943722,7.95365496546363));
#44824=CARTESIAN_POINT('Ctrl Pts',(22.2021924978507,-2.13230602370348,8.65413061376549));
#44825=CARTESIAN_POINT('Ctrl Pts',(22.1723227660645,-2.3833709898048,9.0519012629098));
#44826=CARTESIAN_POINT('Ctrl Pts',(22.1424530342782,-2.51228225890651,9.52677290952939));
#44827=CARTESIAN_POINT('Ctrl Pts',(22.112583302492,-2.51379319101573,10.0008824115804));
#44828=CARTESIAN_POINT('Ctrl Pts',(22.387416697508,-2.52120696757832,9.99913427807354));
#44829=CARTESIAN_POINT('Ctrl Pts',(22.3904924784145,-2.52142393178175,9.9506815244235));
#44830=CARTESIAN_POINT('Ctrl Pts',(22.393568259321,-2.52014729821555,9.90224042487485));
#44831=CARTESIAN_POINT('Ctrl Pts',(22.3966440402275,-2.5173408263703,9.85388812043869));
#44832=CARTESIAN_POINT('Ctrl Pts',(22.4493954767505,-2.46920819732477,9.0246178974504));
#44833=CARTESIAN_POINT('Ctrl Pts',(22.5021469132734,-1.97108510292534,8.22146609138159));
#44834=CARTESIAN_POINT('Ctrl Pts',(22.5548983497963,-1.24958996734608,7.80982228635205));
#44835=CARTESIAN_POINT('Ctrl Pts',(22.6076497863193,-0.528094831766828,
7.39817848132251));
#44836=CARTESIAN_POINT('Ctrl Pts',(22.6604012228422,0.41677234499225,7.37804267733221));
#44837=CARTESIAN_POINT('Ctrl Pts',(22.7131526593651,1.1551493388732,7.75857555916865));
#44838=CARTESIAN_POINT('Ctrl Pts',(22.765904095888,1.89352633275415,8.13910844100509));
#44839=CARTESIAN_POINT('Ctrl Pts',(22.818655532411,2.42541314375697,8.92031000866826));
#44840=CARTESIAN_POINT('Ctrl Pts',(22.8714069689339,2.50883071324478,9.74677679829437));
#44841=CARTESIAN_POINT('Ctrl Pts',(22.9241584054568,2.59224828273258,10.5732435879205));
#44842=CARTESIAN_POINT('Ctrl Pts',(22.9769098419798,2.22719661070537,11.4449755995095));
#44843=CARTESIAN_POINT('Ctrl Pts',(23.0296612785027,1.57975402480848,11.9653830831136));
#44844=CARTESIAN_POINT('Ctrl Pts',(23.0824127150256,0.932311438911595,12.4857905667176));
#44845=CARTESIAN_POINT('Ctrl Pts',(23.1351641515485,0.00247793914503677,
12.6548735223365));
#44846=CARTESIAN_POINT('Ctrl Pts',(23.1879155880715,-0.786723799438258,
12.3957085041788));
#44847=CARTESIAN_POINT('Ctrl Pts',(23.2406670245944,-1.57592553802155,12.1365434860212));
#44848=CARTESIAN_POINT('Ctrl Pts',(23.2934184611173,-2.22449551542159,11.4491304940869));
#44849=CARTESIAN_POINT('Ctrl Pts',(23.3461698976402,-2.4373701819469,10.6462044936153));
#44850=CARTESIAN_POINT('Ctrl Pts',(23.3599188309295,-2.49285302340009,10.4369329221786));
#44851=CARTESIAN_POINT('Ctrl Pts',(23.3736677642188,-2.51873854991203,10.2198144109009));
#44852=CARTESIAN_POINT('Ctrl Pts',(23.387416697508,-2.51682157436921,10.00224693272));
#44853=CARTESIAN_POINT('Origin',(17.,0.,10.));
#44854=CARTESIAN_POINT('',(24.387416697508,-2.51385573226095,9.99896352468483));
#44855=CARTESIAN_POINT('',(24.112583302492,-2.52041830912221,10.0014523913097));
#44856=CARTESIAN_POINT('',(17.,-2.5175,10.));
#44857=CARTESIAN_POINT('Ctrl Pts',(24.112583302492,-2.52041830912221,10.0014523913097));
#44858=CARTESIAN_POINT('Ctrl Pts',(24.1069949230716,-2.5210272662623,10.0895589550511));
#44859=CARTESIAN_POINT('Ctrl Pts',(24.1014065436512,-2.51680247988567,10.1776065034683));
#44860=CARTESIAN_POINT('Ctrl Pts',(24.0958181642308,-2.50754945116842,10.265122427668));
#44861=CARTESIAN_POINT('Ctrl Pts',(24.0432174512758,-2.42045516659928,11.0888674996318));
#44862=CARTESIAN_POINT('Ctrl Pts',(23.9906167383208,-1.88788141364161,11.865513076825));
#44863=CARTESIAN_POINT('Ctrl Pts',(23.9380160253658,-1.15085300692774,12.243575552908));
#44864=CARTESIAN_POINT('Ctrl Pts',(23.8854153124108,-0.413824600213868,
12.6216380289909));
#44865=CARTESIAN_POINT('Ctrl Pts',(23.8328145994558,0.527658460256214,12.6011174039635));
#44866=CARTESIAN_POINT('Ctrl Pts',(23.7802138865008,1.24751435885636,12.1913011667028));
#44867=CARTESIAN_POINT('Ctrl Pts',(23.7276131735458,1.96737025745651,11.7814849294421));
#44868=CARTESIAN_POINT('Ctrl Pts',(23.6750124605908,2.46559899418673,10.982373079948));
#44869=CARTESIAN_POINT('Ctrl Pts',(23.6224117476358,2.51671957482837,10.1556152639013));
#44870=CARTESIAN_POINT('Ctrl Pts',(23.5698110346808,2.56784015547002,9.3288574478546));
#44871=CARTESIAN_POINT('Ctrl Pts',(23.5172103217258,2.17185258002309,8.47445366525525));
#44872=CARTESIAN_POINT('Ctrl Pts',(23.4646096087708,1.50796700170717,7.97907720145607));
#44873=CARTESIAN_POINT('Ctrl Pts',(23.4120088958157,0.844081423391251,7.48370073765689));
#44874=CARTESIAN_POINT('Ctrl Pts',(23.3594081828607,-0.0877021577936639,
7.3473515926579));
#44875=CARTESIAN_POINT('Ctrl Pts',(23.3068074699057,-0.865691280649959,
7.63173651802616));
#44876=CARTESIAN_POINT('Ctrl Pts',(23.2542067569507,-1.64368040350625,7.91612144339442));
#44877=CARTESIAN_POINT('Ctrl Pts',(23.2016060439957,-2.26787506803393,8.62124043912995));
#44878=CARTESIAN_POINT('Ctrl Pts',(23.1490053310407,-2.45578667731971,9.42798146571124));
#44879=CARTESIAN_POINT('Ctrl Pts',(23.1368646548578,-2.499158218715,9.61418391463194));
#44880=CARTESIAN_POINT('Ctrl Pts',(23.1247239786749,-2.51928790251381,9.80580001586207));
#44881=CARTESIAN_POINT('Ctrl Pts',(23.112583302492,-2.51755781857958,9.99777508489969));
#44882=CARTESIAN_POINT('Ctrl Pts',(23.387416697508,-2.51682157436921,10.00224693272));
#44883=CARTESIAN_POINT('Ctrl Pts',(23.4264192007417,-2.51138356378068,9.38505895945965));
#44884=CARTESIAN_POINT('Ctrl Pts',(23.4654217039754,-2.28221214670945,8.76425804178077));
#44885=CARTESIAN_POINT('Ctrl Pts',(23.504424207209,-1.87027955385458,8.30872610392666));
#44886=CARTESIAN_POINT('Ctrl Pts',(23.557175643732,-1.31313490358636,7.69261272371846));
#44887=CARTESIAN_POINT('Ctrl Pts',(23.6099270802549,-0.421666247399317,
7.37882497231092));
#44888=CARTESIAN_POINT('Ctrl Pts',(23.6626785167778,0.398558037255763,7.51011936658926));
#44889=CARTESIAN_POINT('Ctrl Pts',(23.7154299533007,1.21878232191084,7.64141376086759));
#44890=CARTESIAN_POINT('Ctrl Pts',(23.7681813898237,1.96776223503395,8.21779030083179));
#44891=CARTESIAN_POINT('Ctrl Pts',(23.8209328263466,2.30475246126436,8.97702867998691));
#44892=CARTESIAN_POINT('Ctrl Pts',(23.8736842628695,2.64174268749477,9.73626705914203));
#44893=CARTESIAN_POINT('Ctrl Pts',(23.9264356993925,2.56674322683247,10.6783672774881));
#44894=CARTESIAN_POINT('Ctrl Pts',(23.9791871359154,2.1138764852266,11.3747276544192));
#44895=CARTESIAN_POINT('Ctrl Pts',(24.0319385724383,1.66100974362073,12.0710880313502));
#44896=CARTESIAN_POINT('Ctrl Pts',(24.0846900089612,0.830275721071305,12.5217085668663));
#44897=CARTESIAN_POINT('Ctrl Pts',(24.1374414454842,-0.000391089040924892,
12.5215785240049));
#44898=CARTESIAN_POINT('Ctrl Pts',(24.1901928820071,-0.831057899153163,
12.5214484811436));
#44899=CARTESIAN_POINT('Ctrl Pts',(24.24294431853,-1.6616574968282,12.0705678599046));
#44900=CARTESIAN_POINT('Ctrl Pts',(24.295695755053,-2.11430637366214,11.3740688240468));
#44901=CARTESIAN_POINT('Ctrl Pts',(24.326269402538,-2.37665235145929,10.9703923102003));
#44902=CARTESIAN_POINT('Ctrl Pts',(24.356843050023,-2.51204002762718,10.4842095460693));
#44903=CARTESIAN_POINT('Ctrl Pts',(24.387416697508,-2.51385573226095,9.99896352468483));
#44904=CARTESIAN_POINT('Origin',(17.,0.,10.));
#44905=CARTESIAN_POINT('',(25.387416697508,-2.52031926711485,9.99879747833012));
#44906=CARTESIAN_POINT('',(25.112583302492,-2.51369118594155,10.0007624228313));
#44907=CARTESIAN_POINT('',(17.,-2.5175,10.));
#44908=CARTESIAN_POINT('',(25.8782388507408,2.51331533716111,9.85490600980483));
#44909=CARTESIAN_POINT('Ctrl Pts',(25.387416697508,-2.52031926711485,9.99879747833012));
#44910=CARTESIAN_POINT('Ctrl Pts',(25.3927697723502,-2.5208983757328,9.91440472807825));
#44911=CARTESIAN_POINT('Ctrl Pts',(25.3981228471923,-2.51703766949288,9.83006045553805));
#44912=CARTESIAN_POINT('Ctrl Pts',(25.4034759220345,-2.50856460058327,9.74617830516996));
#44913=CARTESIAN_POINT('Ctrl Pts',(25.4562273585574,-2.42506743868645,8.91956854142917));
#44914=CARTESIAN_POINT('Ctrl Pts',(25.5089787950803,-1.89366580395695,8.13783525482216));
#44915=CARTESIAN_POINT('Ctrl Pts',(25.5617302316032,-1.15478948854362,7.75787973679709));
#44916=CARTESIAN_POINT('Ctrl Pts',(25.6144816681262,-0.415913173130291,
7.37792421877201));
#44917=CARTESIAN_POINT('Ctrl Pts',(25.6672331046491,0.530437822966877,7.39974646932889));
#44918=CARTESIAN_POINT('Ctrl Pts',(25.719984541172,1.25072220675159,7.81073417797026));
#44919=CARTESIAN_POINT('Ctrl Pts',(25.772735977695,1.9710065905363,8.22172188661162));
#44920=CARTESIAN_POINT('Ctrl Pts',(25.8254874142179,2.46522436200856,9.02187505333746));
#44921=CARTESIAN_POINT('Ctrl Pts',(25.8782388507408,2.51331533716111,9.85490600980485));
#44922=CARTESIAN_POINT('',(25.9598438343188,-1.44740009951425,12.0606038454663));
#44923=CARTESIAN_POINT('Ctrl Pts',(25.9598438343188,-1.44447502497693,12.0618676369297));
#44924=CARTESIAN_POINT('Ctrl Pts',(25.9680986111512,-1.29612166908485,12.1657990016882));
#44925=CARTESIAN_POINT('Ctrl Pts',(25.9758261020123,-1.13376695951384,12.2552771340403));
#44926=CARTESIAN_POINT('Ctrl Pts',(25.9936363108284,-0.65357955075694,12.454243785592));
#44927=CARTESIAN_POINT('Ctrl Pts',(26.,-0.316315187408128,12.5175));
#44928=CARTESIAN_POINT('Ctrl Pts',(26.,0.316315187408128,12.5175));
#44929=CARTESIAN_POINT('Ctrl Pts',(25.9936363108284,0.65357955075694,12.454243785592));
#44930=CARTESIAN_POINT('Ctrl Pts',(25.9706329474538,1.27378145661654,12.1972618359521));
#44931=CARTESIAN_POINT('Ctrl Pts',(25.954319860997,1.55673560227871,12.0035470409956));
#44932=CARTESIAN_POINT('Ctrl Pts',(25.9236560318941,2.00354770900701,11.5567349342673));
#44933=CARTESIAN_POINT('Ctrl Pts',(25.9073094472621,2.19726198315605,11.2737810818527));
#44934=CARTESIAN_POINT('Ctrl Pts',(25.8842294016963,2.45424354267521,10.6535801565147));
#44935=CARTESIAN_POINT('Ctrl Pts',(25.8778320913866,2.5175,10.3163161332307));
#44936=CARTESIAN_POINT('Ctrl Pts',(25.8778320913866,2.5175,9.95206425392299));
#44937=CARTESIAN_POINT('Ctrl Pts',(25.8779655959498,2.51612889288328,9.90364236848503));
#44938=CARTESIAN_POINT('Ctrl Pts',(25.8782388507408,2.51331533716111,9.85490600980483));
#44939=CARTESIAN_POINT('Ctrl Pts',(25.9598438343188,-1.44740009951425,12.0606038454663));
#44940=CARTESIAN_POINT('Ctrl Pts',(25.9171097867945,-0.891269470133681,
12.4428005051404));
#44941=CARTESIAN_POINT('Ctrl Pts',(25.8743757392702,-0.173138502655974,
12.6040916696052));
#44942=CARTESIAN_POINT('Ctrl Pts',(25.8316416917459,0.487362244993046,12.4744336608074));
#44943=CARTESIAN_POINT('Ctrl Pts',(25.7790409787909,1.30036293756482,12.3148395175376));
#44944=CARTESIAN_POINT('Ctrl Pts',(25.7264402658359,2.02604930930844,11.7144344675171));
#44945=CARTESIAN_POINT('Ctrl Pts',(25.6738395528809,2.33692684617734,10.9464895031126));
#44946=CARTESIAN_POINT('Ctrl Pts',(25.6212388399259,2.64780438304624,10.1785445387081));
#44947=CARTESIAN_POINT('Ctrl Pts',(25.5686381269709,2.54387308504042,9.24305965991953));
#44948=CARTESIAN_POINT('Ctrl Pts',(25.5160374140159,2.07170855144438,8.56261910495375));
#44949=CARTESIAN_POINT('Ctrl Pts',(25.4634367010609,1.59954401784833,7.88217854998797));
#44950=CARTESIAN_POINT('Ctrl Pts',(25.4108359881058,0.759146248662072,7.45678231884493));
#44951=CARTESIAN_POINT('Ctrl Pts',(25.3582352751508,-0.0689135765338292,
7.47935431018827));
#44952=CARTESIAN_POINT('Ctrl Pts',(25.3056345621958,-0.896973401729732,
7.50192630153161));
#44953=CARTESIAN_POINT('Ctrl Pts',(25.2530338492408,-1.71269528293527,7.97246651536133));
#44954=CARTESIAN_POINT('Ctrl Pts',(25.2004331362858,-2.14703481200095,8.67781519460184));
#44955=CARTESIAN_POINT('Ctrl Pts',(25.1711498583546,-2.38883543468551,9.07048898650142));
#44956=CARTESIAN_POINT('Ctrl Pts',(25.1418665804233,-2.51243626586703,9.53593570955259));
#44957=CARTESIAN_POINT('Ctrl Pts',(25.112583302492,-2.51369118594155,10.0007624228313));
#44958=CARTESIAN_POINT('Origin',(28.2084234471774,0.,10.));
#44959=CARTESIAN_POINT('',(8.79157655282254,-3.07807615307783,10.0009342588364));
#44960=CARTESIAN_POINT('',(8.70842344717745,-3.06851316107703,10.0005037120289));
#44961=CARTESIAN_POINT('',(28.2084234471774,-3.0735,10.0000000000003));
#44962=CARTESIAN_POINT('',(8.,0.793799282532897,7.03077704625431));
#44963=CARTESIAN_POINT('Ctrl Pts',(8.70842344717745,-3.06851316107703,10.0005037120289));
#44964=CARTESIAN_POINT('Ctrl Pts',(8.68328804421001,-3.06903018828163,10.4877872520226));
#44965=CARTESIAN_POINT('Ctrl Pts',(8.60540120471965,-2.73029264571413,11.9969233978531));
#44966=CARTESIAN_POINT('Ctrl Pts',(8.47476292870636,-0.372557211312175,
13.6086112664375));
#44967=CARTESIAN_POINT('Ctrl Pts',(8.31650861913757,2.82494041479191,12.281332723926));
#44968=CARTESIAN_POINT('Ctrl Pts',(8.15825430956879,3.44737991946778,8.87067395584943));
#44969=CARTESIAN_POINT('Ctrl Pts',(8.05275143652293,1.7779394739971,7.29387947745118));
#44970=CARTESIAN_POINT('Ctrl Pts',(8.,0.793799282532855,7.0307770462543));
#44971=CARTESIAN_POINT('',(8.,0.,6.9265));
#44972=CARTESIAN_POINT('Origin',(8.,0.,10.));
#44973=CARTESIAN_POINT('',(8.,-0.7937992825328,7.03077704625429));
#44974=CARTESIAN_POINT('Origin',(8.,0.,10.));
#44975=CARTESIAN_POINT('Ctrl Pts',(8.79157655282254,-3.07807615307782,10.0009342588364));
#44976=CARTESIAN_POINT('Ctrl Pts',(8.7889204426769,-3.07827713215033,10.0520138798573));
#44977=CARTESIAN_POINT('Ctrl Pts',(8.73366361957626,-3.05408484518725,11.114459619653));
#44978=CARTESIAN_POINT('Ctrl Pts',(8.62580608352061,-1.83029914535168,13.1291833116438));
#44979=CARTESIAN_POINT('Ctrl Pts',(8.46800394465562,1.61680800983869,13.245137596954));
#44980=CARTESIAN_POINT('Ctrl Pts',(8.31020180579059,3.60054044813756,10.4226504132617));
#44981=CARTESIAN_POINT('Ctrl Pts',(8.15420049090541,2.33978014667001,7.25641897300791));
#44982=CARTESIAN_POINT('Ctrl Pts',(8.0507998889752,0.148780815319225,6.77559856235343));
#44983=CARTESIAN_POINT('Ctrl Pts',(8.,-0.795613156383193,7.02571472931219));
#44984=CARTESIAN_POINT('Origin',(28.2084234471774,0.,10.));
#44985=CARTESIAN_POINT('',(9.79157655282253,-3.06960368404499,10.0017022409322));
#44986=CARTESIAN_POINT('',(9.70842344717744,-3.07437462459256,9.99730908511578));
#44987=CARTESIAN_POINT('',(28.2084234471774,-3.0735,10.0000000000003));
#44988=CARTESIAN_POINT('Ctrl Pts',(9.70842344717744,-3.07437462459256,9.99730908511578));
#44989=CARTESIAN_POINT('Ctrl Pts',(9.66646333001425,-3.06699116075788,10.8067972882056));
#44990=CARTESIAN_POINT('Ctrl Pts',(9.57175177632812,-2.325029441416,12.6459346938779));
#44991=CARTESIAN_POINT('Ctrl Pts',(9.42428878611906,0.772313381832412,13.5456136953941));
#44992=CARTESIAN_POINT('Ctrl Pts',(9.26603447655028,3.39364577165048,11.2850883447562));
#44993=CARTESIAN_POINT('Ctrl Pts',(9.1077801669815,2.92704762252235,7.85513439723516));
#44994=CARTESIAN_POINT('Ctrl Pts',(8.94952585741271,-0.20266861905204,6.37704123220448));
#44995=CARTESIAN_POINT('Ctrl Pts',(8.81640695081136,-2.68045467182773,7.9061860654363));
#44996=CARTESIAN_POINT('Ctrl Pts',(8.73603948073294,-3.06794510809417,9.46512981693207));
#44997=CARTESIAN_POINT('Ctrl Pts',(8.70842344717745,-3.06851316107703,10.0005037120289));
#44998=CARTESIAN_POINT('Ctrl Pts',(9.79157655282253,-3.069603684045,10.0017022409322));
#44999=CARTESIAN_POINT('Ctrl Pts',(9.77119138707358,-3.07161716533022,10.3965250682061));
#45000=CARTESIAN_POINT('Ctrl Pts',(9.69820550836963,-2.81824968568554,11.8076406238949));
#45001=CARTESIAN_POINT('Ctrl Pts',(9.57261891671066,-0.702623662064588,
13.5565683145601));
#45002=CARTESIAN_POINT('Ctrl Pts',(9.41481677784566,2.59166910069841,12.5349881811848));
#45003=CARTESIAN_POINT('Ctrl Pts',(9.25701463898065,3.54016602667422,9.21889196466343));
#45004=CARTESIAN_POINT('Ctrl Pts',(9.09921250011564,1.28435171110455,6.60984400954655));
#45005=CARTESIAN_POINT('Ctrl Pts',(8.94406647139626,-2.07642740645684,7.06150941801092));
#45006=CARTESIAN_POINT('Ctrl Pts',(8.8415211556319,-3.07429701012116,9.04045022629949));
#45007=CARTESIAN_POINT('Ctrl Pts',(8.79157655282254,-3.07807615307782,10.0009342588364));
#45008=CARTESIAN_POINT('Origin',(28.2084234471774,0.,10.));
#45009=CARTESIAN_POINT('',(10.7915765528225,-3.07225467518151,9.99733889552176));
#45010=CARTESIAN_POINT('',(10.7084234471774,-3.07691672930537,10.0019090684753));
#45011=CARTESIAN_POINT('',(28.2084234471774,-3.0735,10.0000000000003));
#45012=CARTESIAN_POINT('Ctrl Pts',(10.7084234471774,-3.07691672930537,10.0019090684753));
#45013=CARTESIAN_POINT('Ctrl Pts',(10.7023900523414,-3.07776457748099,10.1180544945408));
#45014=CARTESIAN_POINT('Ctrl Pts',(10.6436052209824,-3.01920281481477,11.2488245350352));
#45015=CARTESIAN_POINT('Ctrl Pts',(10.5320689531006,-1.61985329993334,13.2471660282134));
#45016=CARTESIAN_POINT('Ctrl Pts',(10.3738146435318,1.83951385849227,13.127969994097));
#45017=CARTESIAN_POINT('Ctrl Pts',(10.215560333963,3.62512807421833,10.1626691840488));
#45018=CARTESIAN_POINT('Ctrl Pts',(10.0573060243942,2.11227555931511,7.04935467956235));
#45019=CARTESIAN_POINT('Ctrl Pts',(9.89905171482542,-1.32251038305822,6.62080587867383));
#45020=CARTESIAN_POINT('Ctrl Pts',(9.78275752241983,-2.96230896709799,8.56533388251318));
#45021=CARTESIAN_POINT('Ctrl Pts',(9.71921476653717,-3.07627350671224,9.78912459212447));
#45022=CARTESIAN_POINT('Ctrl Pts',(9.70842344717744,-3.07437462459256,9.99730908511578));
#45023=CARTESIAN_POINT('Ctrl Pts',(10.7915765528225,-3.07225467518151,9.99733889552176));
#45024=CARTESIAN_POINT('Ctrl Pts',(10.7534623314703,-3.06599829486339,10.7339319007572));
#45025=CARTESIAN_POINT('Ctrl Pts',(10.662747397163,-2.43255612271171,12.4967446704248));
#45026=CARTESIAN_POINT('Ctrl Pts',(10.5194317499007,0.502799430185017,13.5902749971079));
#45027=CARTESIAN_POINT('Ctrl Pts',(10.3616296110357,3.27976499314249,11.5446760958796));
#45028=CARTESIAN_POINT('Ctrl Pts',(10.2038274721707,3.08811778788391,8.10094449581088));
#45029=CARTESIAN_POINT('Ctrl Pts',(10.0460253333057,0.101323344801963,6.37610534685446));
#45030=CARTESIAN_POINT('Ctrl Pts',(9.90860836018963,-2.5794949399918,7.73044878286791));
#45031=CARTESIAN_POINT('Ctrl Pts',(9.82379210002858,-3.06642169366084,9.37774688110278));
#45032=CARTESIAN_POINT('Ctrl Pts',(9.79157655282253,-3.069603684045,10.0017022409322));
#45033=CARTESIAN_POINT('Origin',(28.2084234471774,0.,10.));
#45034=CARTESIAN_POINT('',(11.7915765528225,-3.07791877256789,10.001096933631));
#45035=CARTESIAN_POINT('',(11.7084234471774,-3.06890348767814,10.0010756969218));
#45036=CARTESIAN_POINT('',(28.2084234471774,-3.0735,10.0000000000003));
#45037=CARTESIAN_POINT('Ctrl Pts',(11.7084234471774,-3.06890348767814,10.0010756969218));
#45038=CARTESIAN_POINT('Ctrl Pts',(11.6855653381456,-3.07030490094272,10.4440452179421));
#45039=CARTESIAN_POINT('Ctrl Pts',(11.6099557925909,-2.77375822075196,11.907501720394));
#45040=CARTESIAN_POINT('Ctrl Pts',(11.4815948105133,-0.526448883152259,
13.5903847416995));
#45041=CARTESIAN_POINT('Ctrl Pts',(11.3233405009445,2.72323490185543,12.3983332956597));
#45042=CARTESIAN_POINT('Ctrl Pts',(11.1650861913757,3.49507659867442,9.02406424380673));
#45043=CARTESIAN_POINT('Ctrl Pts',(11.0068318818069,1.08678570881093,6.53778857091659));
#45044=CARTESIAN_POINT('Ctrl Pts',(10.8546109670742,-2.18084464523734,7.17642888325995));
#45045=CARTESIAN_POINT('Ctrl Pts',(10.7551414888643,-3.07035163494491,9.10256682349923));
#45046=CARTESIAN_POINT('Ctrl Pts',(10.7084234471774,-3.07691672930537,10.0019090684753));
#45047=CARTESIAN_POINT('Ctrl Pts',(11.7915765528225,-3.07791877256789,10.001096933631));
#45048=CARTESIAN_POINT('Ctrl Pts',(11.788333988822,-3.07820828582192,10.0634639827233));
#45049=CARTESIAN_POINT('Ctrl Pts',(11.7324907118664,-3.04835338254568,11.137263907321));
#45050=CARTESIAN_POINT('Ctrl Pts',(11.6240467219557,-1.7956016590295,13.1493962879665));
#45051=CARTESIAN_POINT('Ctrl Pts',(11.4662445830908,1.65259091012735,13.2267360548792));
#45052=CARTESIAN_POINT('Ctrl Pts',(11.3084424442257,3.60497432328288,10.3834611087496));
#45053=CARTESIAN_POINT('Ctrl Pts',(11.1506403053608,2.29438831935563,7.19310410595708));
#45054=CARTESIAN_POINT('Ctrl Pts',(10.9928381664957,-1.09291675350356,6.5433520284504));
#45055=CARTESIAN_POINT('Ctrl Pts',(10.873150248983,-2.91177954598531,8.42356662734618));
#45056=CARTESIAN_POINT('Ctrl Pts',(10.8060630444253,-3.07463260650809,9.71737388491982));
#45057=CARTESIAN_POINT('Ctrl Pts',(10.7915765528225,-3.07225467518151,9.99733889552176));
#45058=CARTESIAN_POINT('Origin',(28.2084234471774,0.,10.));
#45059=CARTESIAN_POINT('',(12.7915765528225,-3.06941961343749,10.0015551958711));
#45060=CARTESIAN_POINT('',(12.7084234471775,-3.07305765256541,9.99723902520708));
#45061=CARTESIAN_POINT('',(28.2084234471774,-3.0735,10.0000000000003));
#45062=CARTESIAN_POINT('Ctrl Pts',(12.7084234471775,-3.0730576525654,9.99723902520708));
#45063=CARTESIAN_POINT('Ctrl Pts',(12.6687406239499,-3.06618522061749,10.763633229918));
#45064=CARTESIAN_POINT('Ctrl Pts',(12.5763063641994,-2.38924445855591,12.5596491752114));
#45065=CARTESIAN_POINT('Ctrl Pts',(12.431120667926,0.619461886626625,13.5755108676666));
#45066=CARTESIAN_POINT('Ctrl Pts',(12.2728663583572,3.33534949119645,11.4294945832771));
#45067=CARTESIAN_POINT('Ctrl Pts',(12.1146120487884,3.01643851828712,7.98279657484158));
#45068=CARTESIAN_POINT('Ctrl Pts',(11.9563577392196,-0.047097373778369,
6.37153023510597));
#45069=CARTESIAN_POINT('Ctrl Pts',(11.8209615386826,-2.63147522942551,7.81763283424629));
#45070=CARTESIAN_POINT('Ctrl Pts',(11.7383167746686,-3.0670707505252,9.42176999223617));
#45071=CARTESIAN_POINT('Ctrl Pts',(11.7084234471774,-3.06890348767814,10.0010756969218));
#45072=CARTESIAN_POINT('Ctrl Pts',(12.7915765528225,-3.06941961343749,10.0015551958711));
#45073=CARTESIAN_POINT('Ctrl Pts',(12.7706049332186,-3.07130561059382,10.4077975568445));
#45074=CARTESIAN_POINT('Ctrl Pts',(12.6970326006597,-2.808064557181,11.8306255759708));
#45075=CARTESIAN_POINT('Ctrl Pts',(12.5708595551458,-0.663265918297566,
13.5641212961923));
#45076=CARTESIAN_POINT('Ctrl Pts',(12.4130574162808,2.61953312462283,12.5061780665257));
#45077=CARTESIAN_POINT('Ctrl Pts',(12.2552552774158,3.53131487113802,9.17981857309606));
#45078=CARTESIAN_POINT('Ctrl Pts',(12.0974531385508,1.2467985598852,6.59582966877859));
#45079=CARTESIAN_POINT('Ctrl Pts',(11.9428935636864,-2.09610024567504,7.08283935894699));
#45080=CARTESIAN_POINT('Ctrl Pts',(11.840934701777,-3.07351181612411,9.05174879481766));
#45081=CARTESIAN_POINT('Ctrl Pts',(11.7915765528225,-3.07791877256789,10.001096933631));
#45082=CARTESIAN_POINT('Origin',(28.2084234471774,0.,10.));
#45083=CARTESIAN_POINT('',(13.7915765528225,-3.07257624006984,9.99730578639428));
#45084=CARTESIAN_POINT('',(13.7084234471775,-3.0778195052343,10.0012720431918));
#45085=CARTESIAN_POINT('',(28.2084234471774,-3.0735,10.0000000000003));
#45086=CARTESIAN_POINT('Ctrl Pts',(13.7084234471775,-3.0778195052343,10.0012720431918));
#45087=CARTESIAN_POINT('Ctrl Pts',(13.7046673462771,-3.07819893618978,10.0735226333015));
#45088=CARTESIAN_POINT('Ctrl Pts',(13.6481598088537,-3.04321810478186,11.1601013791998));
#45089=CARTESIAN_POINT('Ctrl Pts',(13.5389008349074,-1.75770622879056,13.1746621562634));
#45090=CARTESIAN_POINT('Ctrl Pts',(13.3806465253387,1.70358963251637,13.2040276773368));
#45091=CARTESIAN_POINT('Ctrl Pts',(13.2223922157699,3.6148076361298,10.3180829245743));
#45092=CARTESIAN_POINT('Ctrl Pts',(13.0641379062011,2.23695110582196,7.14271794474384));
#45093=CARTESIAN_POINT('Ctrl Pts',(12.9058835966323,-1.17628314204709,6.5671631319018));
#45094=CARTESIAN_POINT('Ctrl Pts',(12.7873121102911,-2.93172787836758,8.47620309413993));
#45095=CARTESIAN_POINT('Ctrl Pts',(12.7214920604728,-3.0753209279128,9.74484494941923));
#45096=CARTESIAN_POINT('Ctrl Pts',(12.7084234471775,-3.0730576525654,9.99723902520708));
#45097=CARTESIAN_POINT('Ctrl Pts',(13.7915765528225,-3.07257624006985,9.99730578639428));
#45098=CARTESIAN_POINT('Ctrl Pts',(13.7528758776153,-3.06608888043261,10.7450332734399));
#45099=CARTESIAN_POINT('Ctrl Pts',(13.6615744894531,-2.41686838919438,12.519140261949));
#45100=CARTESIAN_POINT('Ctrl Pts',(13.5176723883359,0.542456216386849,13.5844976699054));
#45101=CARTESIAN_POINT('Ctrl Pts',(13.3598702494708,3.2966397172568,11.5083265120178));
#45102=CARTESIAN_POINT('Ctrl Pts',(13.2020681106059,3.06693661782036,8.06692419328139));
#45103=CARTESIAN_POINT('Ctrl Pts',(13.0442659717408,0.0612580212745303,
6.37520624764731));
#45104=CARTESIAN_POINT('Ctrl Pts',(12.9074354524797,-2.59304903354642,7.75319630627082));
#45105=CARTESIAN_POINT('Ctrl Pts',(12.8232056461736,-3.06657517980556,9.38886634297939));
#45106=CARTESIAN_POINT('Ctrl Pts',(12.7915765528225,-3.06941961343749,10.0015551958711));
#45107=CARTESIAN_POINT('Origin',(28.2084234471774,0.,10.));
#45108=CARTESIAN_POINT('',(14.7915765528225,-3.07773737838628,10.0012785594934));
#45109=CARTESIAN_POINT('',(14.7084234471774,-3.0695085210094,10.001693524509));
#45110=CARTESIAN_POINT('',(28.2084234471774,-3.0735,10.0000000000003));
#45111=CARTESIAN_POINT('Ctrl Pts',(14.7084234471774,-3.0695085210094,10.001693524509));
#45112=CARTESIAN_POINT('Ctrl Pts',(14.6878426320813,-3.07151848242124,10.4003342894936));
#45113=CARTESIAN_POINT('Ctrl Pts',(14.6145103804622,-2.81450704047269,11.8182548620302));
#45114=CARTESIAN_POINT('Ctrl Pts',(14.4884266923202,-0.680037386513999,
13.5644859581834));
#45115=CARTESIAN_POINT('Ctrl Pts',(14.3301723827514,2.61780712972438,12.5129856395747));
#45116=CARTESIAN_POINT('Ctrl Pts',(14.1719180731826,3.53373713437049,9.17494675425479));
#45117=CARTESIAN_POINT('Ctrl Pts',(14.0136637636138,1.23435778144942,6.58761493079715));
#45118=CARTESIAN_POINT('Ctrl Pts',(13.8591655549454,-2.10691859834803,7.09289144011877));
#45119=CARTESIAN_POINT('Ctrl Pts',(13.7574187828,-3.07287013153473,9.05882081378745));
#45120=CARTESIAN_POINT('Ctrl Pts',(13.7084234471775,-3.0778195052343,10.0012720431918));
#45121=CARTESIAN_POINT('Ctrl Pts',(14.7915765528225,-3.07773737838628,10.0012785594934));
#45122=CARTESIAN_POINT('Ctrl Pts',(14.787747534967,-3.07812719640924,10.0749369260762));
#45123=CARTESIAN_POINT('Ctrl Pts',(14.7313178041565,-3.04249024488253,11.1600855874984));
#45124=CARTESIAN_POINT('Ctrl Pts',(14.6222873603909,-1.76067798849733,13.1690527469692));
#45125=CARTESIAN_POINT('Ctrl Pts',(14.4644852215259,1.68815882569895,13.2082708849888));
#45126=CARTESIAN_POINT('Ctrl Pts',(14.3066830826609,3.60899290643803,10.3435876795407));
#45127=CARTESIAN_POINT('Ctrl Pts',(14.1488809437959,2.26322023068206,7.16791305223806));
#45128=CARTESIAN_POINT('Ctrl Pts',(13.9910788049309,-1.13106034981207,6.55564450479696));
#45129=CARTESIAN_POINT('Ctrl Pts',(13.8719773412731,-2.92021801474013,8.44653952308092));
#45130=CARTESIAN_POINT('Ctrl Pts',(13.8054765905703,-3.07490629098906,9.72874612330486));
#45131=CARTESIAN_POINT('Ctrl Pts',(13.7915765528225,-3.07257624006985,9.99730578639428));
#45132=CARTESIAN_POINT('Origin',(28.2084234471774,0.,10.));
#45133=CARTESIAN_POINT('',(15.7915765528225,-3.06925303971756,10.0014017874572));
#45134=CARTESIAN_POINT('',(15.7084234471775,-3.07179824204593,9.99736628792378));
#45135=CARTESIAN_POINT('',(28.2084234471774,-3.0735,10.0000000000003));
#45136=CARTESIAN_POINT('Ctrl Pts',(15.7084234471775,-3.07179824204593,9.99736628792378));
#45137=CARTESIAN_POINT('Ctrl Pts',(15.6710179178855,-3.0658222301893,10.7205329315404));
#45138=CARTESIAN_POINT('Ctrl Pts',(15.5808609520707,-2.45041977337874,12.4727067956687));
#45139=CARTESIAN_POINT('Ctrl Pts',(15.4379525497329,0.465456076952267,13.598800026894));
#45140=CARTESIAN_POINT('Ctrl Pts',(15.2796982401641,3.27093342747344,11.5713069420647));
#45141=CARTESIAN_POINT('Ctrl Pts',(15.1214439305953,3.10022368274011,8.11409859480372));
#45142=CARTESIAN_POINT('Ctrl Pts',(14.9631896210265,0.108653800813268,6.37285162355982));
#45143=CARTESIAN_POINT('Ctrl Pts',(14.8255161265539,-2.57987130069616,7.7291541803051));
#45144=CARTESIAN_POINT('Ctrl Pts',(14.7405940686042,-3.06636667714361,9.37856363020343));
#45145=CARTESIAN_POINT('Ctrl Pts',(14.7084234471774,-3.0695085210094,10.001693524509));
#45146=CARTESIAN_POINT('Ctrl Pts',(15.7915765528225,-3.06925303971756,10.0014017874572));
#45147=CARTESIAN_POINT('Ctrl Pts',(15.7700184793637,-3.0709947854797,10.419061215057));
#45148=CARTESIAN_POINT('Ctrl Pts',(15.6958596929498,-2.79771444910674,11.8536079306759));
#45149=CARTESIAN_POINT('Ctrl Pts',(15.569100193581,-0.623826992014808,13.5712353851694));
#45150=CARTESIAN_POINT('Ctrl Pts',(15.4112980547159,2.6470767906288,12.4770681776581));
#45151=CARTESIAN_POINT('Ctrl Pts',(15.2534959158509,3.52203268603658,9.14083293199628));
#45152=CARTESIAN_POINT('Ctrl Pts',(15.0956937769859,1.20909210531671,6.58225533822185));
#45153=CARTESIAN_POINT('Ctrl Pts',(14.9417206559765,-2.11555602202281,7.10420025525831));
#45154=CARTESIAN_POINT('Ctrl Pts',(14.840348247922,-3.07277211406065,9.06306319147173));
#45155=CARTESIAN_POINT('Ctrl Pts',(14.7915765528225,-3.07773737838628,10.0012785594934));
#45156=CARTESIAN_POINT('Origin',(28.2084234471774,0.,10.));
#45157=CARTESIAN_POINT('',(16.7915765528225,-3.07290364494114,9.99728541773805));
#45158=CARTESIAN_POINT('',(16.7084234471774,-3.07836763528546,10.0005201776737));
#45159=CARTESIAN_POINT('',(28.2084234471774,-3.0735,10.0000000000003));
#45160=CARTESIAN_POINT('Ctrl Pts',(16.7084234471774,-3.07836763528546,10.0005201776737));
#45161=CARTESIAN_POINT('Ctrl Pts',(16.7069446402127,-3.07843463866697,10.0289523017141));
#45162=CARTESIAN_POINT('Ctrl Pts',(16.652714396725,-3.06523049811435,11.0715405015603));
#45163=CARTESIAN_POINT('Ctrl Pts',(16.5457327167144,-1.89232070283748,13.0963096341866));
#45164=CARTESIAN_POINT('Ctrl Pts',(16.3874784071456,1.56452653085165,13.2741819936291));
#45165=CARTESIAN_POINT('Ctrl Pts',(16.2292240975768,3.59782792524174,10.4729114224616));
#45166=CARTESIAN_POINT('Ctrl Pts',(16.070969788008,2.35750444175658,7.24134384160661));
#45167=CARTESIAN_POINT('Ctrl Pts',(15.9127154784392,-1.02788694119381,6.51984778648015));
#45168=CARTESIAN_POINT('Ctrl Pts',(15.7918666981624,-2.89889441257722,8.38698272986147));
#45169=CARTESIAN_POINT('Ctrl Pts',(15.7237693544085,-3.07424994705583,9.70068158821311));
#45170=CARTESIAN_POINT('Ctrl Pts',(15.7084234471775,-3.07179824204593,9.99736628792378));
#45171=CARTESIAN_POINT('Ctrl Pts',(16.7915765528225,-3.07290364494114,9.99728541773805));
#45172=CARTESIAN_POINT('Ctrl Pts',(16.7522894237604,-3.0662073138402,10.7561373882069));
#45173=CARTESIAN_POINT('Ctrl Pts',(16.6604015817432,-2.4009813074848,12.541494677525));
#45174=CARTESIAN_POINT('Ctrl Pts',(16.515913026771,0.582046717903019,13.5782822569538));
#45175=CARTESIAN_POINT('Ctrl Pts',(16.358110887906,3.3131115922785,11.4717927399475));
#45176=CARTESIAN_POINT('Ctrl Pts',(16.200308749041,3.04538068264102,8.03313986515331));
#45177=CARTESIAN_POINT('Ctrl Pts',(16.042506610176,0.0211851935724078,6.37475056308874));
#45178=CARTESIAN_POINT('Ctrl Pts',(15.9062625447698,-2.60641680486434,7.77596614521566));
#45179=CARTESIAN_POINT('Ctrl Pts',(15.8226191923187,-3.06674500550516,9.39999131968569));
#45180=CARTESIAN_POINT('Ctrl Pts',(15.7915765528225,-3.06925303971756,10.0014017874572));
#45181=CARTESIAN_POINT('Origin',(28.2084234471774,0.,10.));
#45182=CARTESIAN_POINT('',(17.7915765528225,-3.07753293276637,10.0014524138578));
#45183=CARTESIAN_POINT('',(17.7084234471775,-3.07037063174865,10.0022000552251));
#45184=CARTESIAN_POINT('',(28.2084234471774,-3.0735,10.0000000000003));
#45185=CARTESIAN_POINT('Ctrl Pts',(17.7084234471775,-3.07037063174865,10.0022000552251));
#45186=CARTESIAN_POINT('Ctrl Pts',(17.6901199260169,-3.07273452913448,10.3564806138557));
#45187=CARTESIAN_POINT('Ctrl Pts',(17.6190649683335,-2.85277747528598,11.7289669017069));
#45188=CARTESIAN_POINT('Ctrl Pts',(17.4952585741271,-0.832373015781326,
13.5320201239153));
#45189=CARTESIAN_POINT('Ctrl Pts',(17.3370042645583,2.50755641786257,12.6230081594193));
#45190=CARTESIAN_POINT('Ctrl Pts',(17.1787499549895,3.56588727515458,9.32734932243063));
#45191=CARTESIAN_POINT('Ctrl Pts',(17.0204956454207,1.37965570806092,6.64372809201059));
#45192=CARTESIAN_POINT('Ctrl Pts',(16.8637201428167,-2.02975002902867,7.01048305338277));
#45193=CARTESIAN_POINT('Ctrl Pts',(16.7596960767356,-3.07604451966515,9.0147324459357));
#45194=CARTESIAN_POINT('Ctrl Pts',(16.7084234471774,-3.07836763528546,10.0005201776737));
#45195=CARTESIAN_POINT('Ctrl Pts',(17.7915765528225,-3.07753293276637,10.0014524138578));
#45196=CARTESIAN_POINT('Ctrl Pts',(17.787161081112,-3.07803302068731,10.0864072843152));
#45197=CARTESIAN_POINT('Ctrl Pts',(17.7301448964466,-3.03649421916237,11.1829179356957));
#45198=CARTESIAN_POINT('Ctrl Pts',(17.6205279988261,-1.72553916596101,13.1883219534713));
#45199=CARTESIAN_POINT('Ctrl Pts',(17.462725859961,1.72352045101636,13.1894136682438));
#45200=CARTESIAN_POINT('Ctrl Pts',(17.3049237210961,3.61257047634171,10.3036722669531));
#45201=CARTESIAN_POINT('Ctrl Pts',(17.147121582231,2.23177558030935,7.14306807022165));
#45202=CARTESIAN_POINT('Ctrl Pts',(16.989319443366,-1.1690657327204,6.56835788508897));
#45203=CARTESIAN_POINT('Ctrl Pts',(16.8708044335632,-2.92850548206875,8.46950746821872));
#45204=CARTESIAN_POINT('Ctrl Pts',(16.8048901367154,-3.07517289107886,9.74012640377492));
#45205=CARTESIAN_POINT('Ctrl Pts',(16.7915765528225,-3.07290364494114,9.99728541773805));
#45206=CARTESIAN_POINT('Origin',(28.2084234471774,0.,10.));
#45207=CARTESIAN_POINT('',(18.7915765528225,-3.06910451058797,10.0012422495348));
#45208=CARTESIAN_POINT('',(18.7084234471775,-3.07067170632208,9.99767573393063));
#45209=CARTESIAN_POINT('',(28.2084234471774,-3.0735,10.0000000000003));
#45210=CARTESIAN_POINT('Ctrl Pts',(18.7084234471775,-3.07067170632208,9.99767573393063));
#45211=CARTESIAN_POINT('Ctrl Pts',(18.6732952118212,-3.06584729530095,10.6774452904515));
#45212=CARTESIAN_POINT('Ctrl Pts',(18.585415539942,-2.50862065342642,12.3851967347818));
#45213=CARTESIAN_POINT('Ctrl Pts',(18.4447844315398,0.31059273116958,13.6154589125709));
#45214=CARTESIAN_POINT('Ctrl Pts',(18.286530121971,3.2004911372734,11.7102243926977));
#45215=CARTESIAN_POINT('Ctrl Pts',(18.1282758124023,3.17829712925949,8.24887511830688));
#45216=CARTESIAN_POINT('Ctrl Pts',(17.9700215028334,0.264204795973602,6.38085551284168));
#45217=CARTESIAN_POINT('Ctrl Pts',(17.8300707144252,-2.52543982199027,7.64104243304114));
#45218=CARTESIAN_POINT('Ctrl Pts',(17.7428713625399,-3.06592168794387,9.33543071662528));
#45219=CARTESIAN_POINT('Ctrl Pts',(17.7084234471775,-3.07037063174865,10.0022000552251));
#45220=CARTESIAN_POINT('Ctrl Pts',(18.7915765528225,-3.06910451058797,10.0012422495348));
#45221=CARTESIAN_POINT('Ctrl Pts',(18.7694320255087,-3.07068542358524,10.4303154839391));
#45222=CARTESIAN_POINT('Ctrl Pts',(18.6946867852399,-2.78719815131979,11.8765861322557));
#45223=CARTESIAN_POINT('Ctrl Pts',(18.5673408320161,-0.584311835073177,
13.5779130749147));
#45224=CARTESIAN_POINT('Ctrl Pts',(18.4095386931511,2.6742969880911,12.4476555950008));
#45225=CARTESIAN_POINT('Ctrl Pts',(18.2517365542861,3.51232011417934,9.10195227978501));
#45226=CARTESIAN_POINT('Ctrl Pts',(18.0939344154211,1.17123790163294,6.56909865049566));
#45227=CARTESIAN_POINT('Ctrl Pts',(17.9405477482666,-2.13479723191698,7.12563505721765));
#45228=CARTESIAN_POINT('Ctrl Pts',(17.8397617940671,-3.07207556406519,9.07435533425115));
#45229=CARTESIAN_POINT('Ctrl Pts',(17.7915765528225,-3.07753293276637,10.0014524138578));
#45230=CARTESIAN_POINT('Origin',(28.2084234471774,0.,10.));
#45231=CARTESIAN_POINT('',(19.7915765528226,-3.07323555454232,9.99727800514525));
#45232=CARTESIAN_POINT('',(19.7084234471775,-3.07844518169678,9.99971767584083));
#45233=CARTESIAN_POINT('',(28.2084234471774,-3.0735,10.0000000000003));
#45234=CARTESIAN_POINT('Ctrl Pts',(19.7084234471775,-3.07844518169678,9.99971767584083));
#45235=CARTESIAN_POINT('Ctrl Pts',(19.6564704976254,-3.07712673515848,10.9985178159267));
#45236=CARTESIAN_POINT('Ctrl Pts',(19.5517661115504,-2.00606157994286,13.0138977284695));
#45237=CARTESIAN_POINT('Ctrl Pts',(19.3943102889525,1.42258101312554,13.3383040985265));
#45238=CARTESIAN_POINT('Ctrl Pts',(19.2360559793837,3.57421973167857,10.6268686487801));
#45239=CARTESIAN_POINT('Ctrl Pts',(19.0778016698149,2.47371441340158,7.34505216735374));
#45240=CARTESIAN_POINT('Ctrl Pts',(18.9195473602461,-0.877597005871997,
6.47894412307493));
#45241=CARTESIAN_POINT('Ctrl Pts',(18.7964212860336,-2.86373988760194,8.297708117217));
#45242=CARTESIAN_POINT('Ctrl Pts',(18.7260466483441,-3.07309202618938,9.65664762591398));
#45243=CARTESIAN_POINT('Ctrl Pts',(18.7084234471775,-3.07067170632208,9.99767573393063));
#45244=CARTESIAN_POINT('Ctrl Pts',(19.7915765528226,-3.07323555454232,9.99727800514525));
#45245=CARTESIAN_POINT('Ctrl Pts',(19.7517029699054,-3.06635454716845,10.7672451060908));
#45246=CARTESIAN_POINT('Ctrl Pts',(19.6592286740333,-2.38489386469174,12.5638062052433));
#45247=CARTESIAN_POINT('Ctrl Pts',(19.5141536652062,0.621566094242422,13.5716295836412));
#45248=CARTESIAN_POINT('Ctrl Pts',(19.3563515263411,3.32917861036942,11.4350791171607));
#45249=CARTESIAN_POINT('Ctrl Pts',(19.1985493874761,3.02345260681924,7.99959588418488));
#45250=CARTESIAN_POINT('Ctrl Pts',(19.0407472486111,-0.0188902229263912,
6.37473787820383));
#45251=CARTESIAN_POINT('Ctrl Pts',(18.9050896370599,-2.61959942140483,7.79875770460526));
#45252=CARTESIAN_POINT('Ctrl Pts',(18.8220327384637,-3.06693022260047,9.4111219956457));
#45253=CARTESIAN_POINT('Ctrl Pts',(18.7915765528225,-3.06910451058797,10.0012422495348));
#45254=CARTESIAN_POINT('Origin',(28.2084234471774,0.,10.));
#45255=CARTESIAN_POINT('',(20.7915765528225,-3.07730739150996,10.0016176250368));
#45256=CARTESIAN_POINT('',(20.7084234471775,-3.0714446790292,10.0025593696137));
#45257=CARTESIAN_POINT('',(28.2084234471774,-3.0735,10.0000000000003));
#45258=CARTESIAN_POINT('Ctrl Pts',(20.7084234471775,-3.0714446790292,10.0025593696137));
#45259=CARTESIAN_POINT('Ctrl Pts',(20.6923972199526,-3.07391157156986,10.3124871628441));
#45260=CARTESIAN_POINT('Ctrl Pts',(20.6236195562048,-2.88863851193006,11.6396831302958));
#45261=CARTESIAN_POINT('Ctrl Pts',(20.502090455934,-0.983175116979502,13.4930470484227));
#45262=CARTESIAN_POINT('Ctrl Pts',(20.3438361463652,2.39268589243202,12.7281981623963));
#45263=CARTESIAN_POINT('Ctrl Pts',(20.1855818367964,3.59146777933862,9.48099115314302));
#45264=CARTESIAN_POINT('Ctrl Pts',(20.0273275272277,1.52241181662405,6.70602470353113));
#45265=CARTESIAN_POINT('Ctrl Pts',(19.8690732176588,-1.93187026052108,6.9282108975943));
#45266=CARTESIAN_POINT('Ctrl Pts',(19.7627718576421,-3.07142617074966,8.95488367414853));
#45267=CARTESIAN_POINT('Ctrl Pts',(19.7092219341483,-3.0784654454622,9.9843666918209));
#45268=CARTESIAN_POINT('Ctrl Pts',(19.7084234471775,-3.07844518169678,9.99971767584083));
#45269=CARTESIAN_POINT('Ctrl Pts',(20.7915765528225,-3.07730739150996,10.0016176250368));
#45270=CARTESIAN_POINT('Ctrl Pts',(20.7865746272571,-3.07792592522714,10.0978746732603));
#45271=CARTESIAN_POINT('Ctrl Pts',(20.7289719887367,-3.03036433852053,11.2057607933903));
#45272=CARTESIAN_POINT('Ctrl Pts',(20.6187686372612,-1.69018948530375,13.2072015521334));
#45273=CARTESIAN_POINT('Ctrl Pts',(20.4609664983962,1.75867146489572,13.1701667102578));
#45274=CARTESIAN_POINT('Ctrl Pts',(20.3031643595312,3.61570659591804,10.2637197460999));
#45275=CARTESIAN_POINT('Ctrl Pts',(20.1453622206662,2.20005821053506,7.11857220071228));
#45276=CARTESIAN_POINT('Ctrl Pts',(19.9875600818011,-1.20692825766852,6.58149060655154));
#45277=CARTESIAN_POINT('Ctrl Pts',(19.8696315258533,-2.93664307613956,8.49246995470104));
#45278=CARTESIAN_POINT('Ctrl Pts',(19.8043036828604,-3.07543188276848,9.75151450205139));
#45279=CARTESIAN_POINT('Ctrl Pts',(19.7915765528226,-3.07323555454232,9.99727800514525));
#45280=CARTESIAN_POINT('Origin',(28.2084234471774,0.,10.));
#45281=CARTESIAN_POINT('',(21.7915765528225,-3.06897452734334,10.0010772957271));
#45282=CARTESIAN_POINT('',(21.7084234471775,-3.06974091379035,9.99814174205166));
#45283=CARTESIAN_POINT('',(28.2084234471774,-3.0735,10.0000000000003));
#45284=CARTESIAN_POINT('Ctrl Pts',(21.7084234471775,-3.06974091379035,9.99814174205167));
#45285=CARTESIAN_POINT('Ctrl Pts',(21.6755725057568,-3.0662040854976,10.6343282548533));
#45286=CARTESIAN_POINT('Ctrl Pts',(21.5899701278132,-2.56390958624238,12.2972104532282));
#45287=CARTESIAN_POINT('Ctrl Pts',(21.4516163133467,0.155157162744094,13.6254568329877));
#45288=CARTESIAN_POINT('Ctrl Pts',(21.2933620037779,3.1241524005353,11.845990999834));
#45289=CARTESIAN_POINT('Ctrl Pts',(21.1351076942091,3.2505150185073,8.38687783860446));
#45290=CARTESIAN_POINT('Ctrl Pts',(20.9768533846404,0.419269031639233,6.39552715751162));
#45291=CARTESIAN_POINT('Ctrl Pts',(20.8346253022964,-2.46811551266869,7.55338081248407));
#45292=CARTESIAN_POINT('Ctrl Pts',(20.7451486564755,-3.06579162397138,9.29233837287249));
#45293=CARTESIAN_POINT('Ctrl Pts',(20.7084234471775,-3.0714446790292,10.0025593696137));
#45294=CARTESIAN_POINT('Ctrl Pts',(21.7915765528226,-3.06897452734334,10.0010772957271));
#45295=CARTESIAN_POINT('Ctrl Pts',(21.7688455716538,-3.07037829602215,10.4415604023203));
#45296=CARTESIAN_POINT('Ctrl Pts',(21.69351387753,-2.77651448008785,11.8995593015108));
#45297=CARTESIAN_POINT('Ctrl Pts',(21.5655814704513,-0.544725276252224,
13.5841535492561));
#45298=CARTESIAN_POINT('Ctrl Pts',(21.4077793315862,2.70119039079158,12.4179439128307));
#45299=CARTESIAN_POINT('Ctrl Pts',(21.2499771927212,3.50217834240436,9.06318136752485));
#45300=CARTESIAN_POINT('Ctrl Pts',(21.0921750538562,1.13324057456603,6.55636121344182));
#45301=CARTESIAN_POINT('Ctrl Pts',(20.9393748405567,-2.15382461611422,7.14714164828928));
#45302=CARTESIAN_POINT('Ctrl Pts',(20.8391753402121,-3.07142136731547,9.0856266305313));
#45303=CARTESIAN_POINT('Ctrl Pts',(20.7915765528225,-3.07730739150996,10.0016176250368));
#45304=CARTESIAN_POINT('Origin',(28.2084234471774,0.,10.));
#45305=CARTESIAN_POINT('',(22.7915765528226,-3.07357058804542,9.99728370345179));
#45306=CARTESIAN_POINT('',(22.7084234471774,-3.07802566627685,9.99894307990421));
#45307=CARTESIAN_POINT('',(28.2084234471774,-3.0735,10.0000000000003));
#45308=CARTESIAN_POINT('Ctrl Pts',(22.7084234471774,-3.07802566627685,9.99894307990421));
#45309=CARTESIAN_POINT('Ctrl Pts',(22.658747791561,-3.07374767361358,10.9543104693303));
#45310=CARTESIAN_POINT('Ctrl Pts',(22.5563206994218,-2.08420676059476,12.9318512556298));
#45311=CARTESIAN_POINT('Ctrl Pts',(22.4011421707594,1.27801459267746,13.39627585532));
#45312=CARTESIAN_POINT('Ctrl Pts',(22.2428878611907,3.5440265506493,10.7796709598669));
#45313=CARTESIAN_POINT('Ctrl Pts',(22.0846335516218,2.58536692026875,7.45365185399615));
#45314=CARTESIAN_POINT('Ctrl Pts',(21.9263792420531,-0.725690223623306,
6.44452750096693));
#45315=CARTESIAN_POINT('Ctrl Pts',(21.8009758739049,-2.82619643473853,8.2084169339104));
#45316=CARTESIAN_POINT('Ctrl Pts',(21.7283239422797,-3.07188345921138,9.61275167301163));
#45317=CARTESIAN_POINT('Ctrl Pts',(21.7084234471775,-3.06974091379035,9.99814174205167));
#45318=CARTESIAN_POINT('Ctrl Pts',(22.7915765528226,-3.07357058804542,9.99728370345179));
#45319=CARTESIAN_POINT('Ctrl Pts',(22.7511165160505,-3.06653153385114,10.7783573196862));
#45320=CARTESIAN_POINT('Ctrl Pts',(22.6580557663234,-2.36860505410454,12.5860731442903));
#45321=CARTESIAN_POINT('Ctrl Pts',(22.5123943036413,0.661009511544134,13.5645404549472));
#45322=CARTESIAN_POINT('Ctrl Pts',(22.3545921647763,3.34483881058325,11.3981901341401));
#45323=CARTESIAN_POINT('Ctrl Pts',(22.1967900259113,3.0011550686756,7.96629634724844));
#45324=CARTESIAN_POINT('Ctrl Pts',(22.0389878870462,-0.0589633304184637,
6.37516819565949));
#45325=CARTESIAN_POINT('Ctrl Pts',(21.90391672935,-2.63259802844919,7.82156968830812));
#45326=CARTESIAN_POINT('Ctrl Pts',(21.8214462846088,-3.06712989980111,9.42225880335216));
#45327=CARTESIAN_POINT('Ctrl Pts',(21.7915765528226,-3.06897452734334,10.0010772957271));
#45328=CARTESIAN_POINT('Origin',(28.2084234471774,0.,10.));
#45329=CARTESIAN_POINT('',(23.7915765528225,-3.07706282942884,10.001773157772));
#45330=CARTESIAN_POINT('',(23.7084234471775,-3.07267174134012,10.002743176848));
#45331=CARTESIAN_POINT('',(28.2084234471774,-3.0735,10.0000000000003));
#45332=CARTESIAN_POINT('Ctrl Pts',(23.7084234471775,-3.07267174134012,10.002743176848));
#45333=CARTESIAN_POINT('Ctrl Pts',(23.6946745138882,-3.07501208864137,10.2683613076082));
#45334=CARTESIAN_POINT('Ctrl Pts',(23.628174144076,-2.92215844456484,11.5504428457205));
#45335=CARTESIAN_POINT('Ctrl Pts',(23.5089223377409,-1.13216576586705,13.447638623633));
#45336=CARTESIAN_POINT('Ctrl Pts',(23.3506680281721,2.27340713764739,12.8283618044535));
#45337=CARTESIAN_POINT('Ctrl Pts',(23.1924137186033,3.61043154357666,9.63558920748943));
#45338=CARTESIAN_POINT('Ctrl Pts',(23.0341594090345,1.66236308643603,6.77438998022499));
#45339=CARTESIAN_POINT('Ctrl Pts',(22.8759050994658,-1.79827159213679,6.848138612079));
#45340=CARTESIAN_POINT('Ctrl Pts',(22.7673264455134,-3.05000135332916,8.86637271869838));
#45341=CARTESIAN_POINT('Ctrl Pts',(22.7114992280839,-3.07829054789721,9.93978934074102));
#45342=CARTESIAN_POINT('Ctrl Pts',(22.7084234471774,-3.07802566627685,9.99894307990421));
#45343=CARTESIAN_POINT('Ctrl Pts',(23.7915765528225,-3.07706282942884,10.001773157772));
#45344=CARTESIAN_POINT('Ctrl Pts',(23.7859881734021,-3.07780627720245,10.1093384104667));
#45345=CARTESIAN_POINT('Ctrl Pts',(23.7277990810267,-3.02410010614128,11.2286131560421));
#45346=CARTESIAN_POINT('Ctrl Pts',(23.6170092756964,-1.65463280838614,13.2256900191163));
#45347=CARTESIAN_POINT('Ctrl Pts',(23.4592071368313,1.79360733424122,13.1505319563297));
#45348=CARTESIAN_POINT('Ctrl Pts',(23.3014049979663,3.61840100535183,10.2237352102483));
#45349=CARTESIAN_POINT('Ctrl Pts',(23.1436028591013,2.16807193309428,7.09442832744505));
#45350=CARTESIAN_POINT('Ctrl Pts',(22.9858007202363,-1.24464326464773,6.59504112130271));
#45351=CARTESIAN_POINT('Ctrl Pts',(22.8684586181434,-2.94463192189129,8.5154264800344));
#45352=CARTESIAN_POINT('Ctrl Pts',(22.8037172290055,-3.07568276797467,9.76291016832276));
#45353=CARTESIAN_POINT('Ctrl Pts',(22.7915765528226,-3.07357058804542,9.99728370345179));
#45354=CARTESIAN_POINT('Origin',(28.2084234471774,0.,10.));
#45355=CARTESIAN_POINT('',(24.7915765528225,-3.06884999403827,10.0009308069803));
#45356=CARTESIAN_POINT('',(24.7084234471775,-3.06905088107409,9.99873461494295));
#45357=CARTESIAN_POINT('',(28.2084234471774,-3.0735,10.0000000000003));
#45358=CARTESIAN_POINT('Ctrl Pts',(24.7084234471775,-3.06905088107409,9.99873461494295));
#45359=CARTESIAN_POINT('Ctrl Pts',(24.6778497996924,-3.06683417076947,10.5911491717355));
#45360=CARTESIAN_POINT('Ctrl Pts',(24.5945247156845,-2.6163584606915,12.2088261427766));
#45361=CARTESIAN_POINT('Ctrl Pts',(24.4584481951536,-0.000559519202797285,
13.6287799388967));
#45362=CARTESIAN_POINT('Ctrl Pts',(24.3001938855848,3.04205539834121,11.9783542595615));
#45363=CARTESIAN_POINT('Ctrl Pts',(24.141939576016,3.31674557789901,8.52785373790922));
#45364=CARTESIAN_POINT('Ctrl Pts',(23.9836852664473,0.573560160241939,6.41683888716847));
#45365=CARTESIAN_POINT('Ctrl Pts',(23.8391798901677,-2.40783492161846,7.46625913576792));
#45366=CARTESIAN_POINT('Ctrl Pts',(23.7474259504111,-3.06603272424225,9.24924675745743));
#45367=CARTESIAN_POINT('Ctrl Pts',(23.7084234471775,-3.07267174134012,10.002743176848));
#45368=CARTESIAN_POINT('Ctrl Pts',(24.7915765528225,-3.06884999403827,10.0009308069803));
#45369=CARTESIAN_POINT('Ctrl Pts',(24.7682591177988,-3.07006994083386,10.4528032974328));
#45370=CARTESIAN_POINT('Ctrl Pts',(24.6923409698201,-2.76569457382785,11.9224712354734));
#45371=CARTESIAN_POINT('Ctrl Pts',(24.5638221088864,-0.505048782495192,
13.5899960272459));
#45372=CARTESIAN_POINT('Ctrl Pts',(24.4060199700213,2.72774157840345,12.387916003312));
#45373=CARTESIAN_POINT('Ctrl Pts',(24.2482178311564,3.49161491002287,9.0245357108578));
#45374=CARTESIAN_POINT('Ctrl Pts',(24.0904156922914,1.09510149634942,6.54403898763965));
#45375=CARTESIAN_POINT('Ctrl Pts',(23.9382019328468,-2.17263741343222,7.16872054184951));
#45376=CARTESIAN_POINT('Ctrl Pts',(23.8385888863571,-3.07080856283935,9.09687870519458));
#45377=CARTESIAN_POINT('Ctrl Pts',(23.7915765528225,-3.07706282942884,10.001773157772));
#45378=CARTESIAN_POINT('Origin',(28.2084234471774,0.,10.));
#45379=CARTESIAN_POINT('',(25.7915765528225,-3.07002684332744,10.000064028751));
#45380=CARTESIAN_POINT('',(25.7084234471775,-3.07694191359583,9.99853189658296));
#45381=CARTESIAN_POINT('',(28.2084234471774,-3.0735,10.0000000000003));
#45382=CARTESIAN_POINT('',(25.8262392198064,-3.00089449353541,9.33589572455161));
#45383=CARTESIAN_POINT('Ctrl Pts',(25.8262392198064,-3.0008944935354,9.33589572455155));
#45384=CARTESIAN_POINT('Ctrl Pts',(25.8146849974785,-3.04910668411157,9.55375262228589));
#45385=CARTESIAN_POINT('Ctrl Pts',(25.8031307751505,-3.07166211508236,9.77686471172983));
#45386=CARTESIAN_POINT('Ctrl Pts',(25.7915765528226,-3.07002654794609,10.0000640341964));
#45387=CARTESIAN_POINT('',(26.,1.26217744835362E-28,6.9265));
#45388=CARTESIAN_POINT('Ctrl Pts',(26.,-2.4980018054066E-15,6.9265));
#45389=CARTESIAN_POINT('Ctrl Pts',(26.,-0.386302212465491,6.9265));
#45390=CARTESIAN_POINT('Ctrl Pts',(25.9905104526593,-0.79810794837382,7.00377648233523));
#45391=CARTESIAN_POINT('Ctrl Pts',(25.9562094606332,-1.55524928118873,7.31755124766488));
#45392=CARTESIAN_POINT('Ctrl Pts',(25.9318826712469,-1.9006150067912,7.55402962283749));
#45393=CARTESIAN_POINT('Ctrl Pts',(25.8861371643816,-2.44597219633851,8.0993868123848));
#45394=CARTESIAN_POINT('Ctrl Pts',(25.8617357704543,-2.68244914732635,8.4447517454274));
#45395=CARTESIAN_POINT('Ctrl Pts',(25.8369342606554,-2.90820005126638,8.98949060270564));
#45396=CARTESIAN_POINT('Ctrl Pts',(25.8307130606305,-2.96239181255062,9.16191328290026));
#45397=CARTESIAN_POINT('Ctrl Pts',(25.8262392198064,-3.00089449353541,9.33589572455161));
#45398=CARTESIAN_POINT('',(25.9920223077014,0.645410697669269,6.99640220569977));
#45399=CARTESIAN_POINT('Ctrl Pts',(25.9920223077014,0.644031331499173,6.99473364008323));
#45400=CARTESIAN_POINT('Ctrl Pts',(25.9973703299551,0.428194140166751,6.94847953243578));
#45401=CARTESIAN_POINT('Ctrl Pts',(26.,0.210221720574735,6.9265));
#45402=CARTESIAN_POINT('Ctrl Pts',(26.,-2.42861286636753E-15,6.9265));
#45403=CARTESIAN_POINT('Ctrl Pts',(25.9920223077014,0.647043985098389,6.99837792998922));
#45404=CARTESIAN_POINT('Ctrl Pts',(25.9555938655585,-0.0431691754597013,
6.85594805878722));
#45405=CARTESIAN_POINT('Ctrl Pts',(25.8664139868927,-1.86387412312115,7.06750307061891));
#45406=CARTESIAN_POINT('Ctrl Pts',(25.7718810333847,-3.02648815522162,8.77779906703974));
#45407=CARTESIAN_POINT('Ctrl Pts',(25.7137765220196,-3.07764892068114,9.89550066802324));
#45408=CARTESIAN_POINT('Ctrl Pts',(25.7084234471775,-3.07694191359583,9.99853189658296));
#45409=CARTESIAN_POINT('Origin',(0.,0.,181.5));
#45410=CARTESIAN_POINT('',(-19.,-2.32682891837997E-15,181.));
#45411=CARTESIAN_POINT('Origin',(0.,0.,181.));
#45412=CARTESIAN_POINT('',(-19.,-2.32682891837997E-15,182.));
#45413=CARTESIAN_POINT('',(-19.,-2.32682891837997E-15,181.5));
#45414=CARTESIAN_POINT('Origin',(0.,0.,182.));
#45415=CARTESIAN_POINT('Origin',(23.,0.,181.));
#45416=CARTESIAN_POINT('',(-20.,2.44929359829471E-15,181.));
#45417=CARTESIAN_POINT('Origin',(0.,0.,181.));
#45418=CARTESIAN_POINT('Origin',(19.,0.,182.));
#45419=CARTESIAN_POINT('',(-20.,-2.44929359829471E-15,182.));
#45420=CARTESIAN_POINT('Origin',(0.,0.,182.));
#45421=CARTESIAN_POINT('Origin',(0.,0.,20.));
#45422=CARTESIAN_POINT('',(-20.,-2.44929359829471E-15,225.));
#45423=CARTESIAN_POINT('Origin',(0.,0.,225.));
#45424=CARTESIAN_POINT('',(-20.,-2.44929359829471E-15,20.));
#45425=CARTESIAN_POINT('Origin',(12.,-4.,240.));
#45426=CARTESIAN_POINT('',(11.3137084989848,-4.,225.));
#45427=CARTESIAN_POINT('',(11.3137084989848,-4.,255.));
#45428=CARTESIAN_POINT('',(11.3137084989848,-4.,220.));
#45429=CARTESIAN_POINT('',(8.,-4.,225.));
#45430=CARTESIAN_POINT('',(8.,-4.,225.));
#45431=CARTESIAN_POINT('',(8.,-4.,255.));
#45432=CARTESIAN_POINT('',(8.,-4.,255.));
#45433=CARTESIAN_POINT('',(16.,-4.,255.));
#45434=CARTESIAN_POINT('Origin',(8.,0.,225.));
#45435=CARTESIAN_POINT('',(8.,4.,255.));
#45436=CARTESIAN_POINT('',(8.,0.,255.));
#45437=CARTESIAN_POINT('',(8.,4.,225.));
#45438=CARTESIAN_POINT('',(8.,0.,225.));
#45439=CARTESIAN_POINT('',(8.,4.,255.));
#45440=CARTESIAN_POINT('Origin',(8.,0.,255.));
#45441=CARTESIAN_POINT('',(11.3137084989848,4.,255.));
#45442=CARTESIAN_POINT('Origin',(0.,0.,255.));
#45443=CARTESIAN_POINT('',(16.,4.,255.));
#45444=CARTESIAN_POINT('Origin',(12.,4.,240.));
#45445=CARTESIAN_POINT('',(11.3137084989848,4.,225.));
#45446=CARTESIAN_POINT('',(11.3137084989848,4.,220.));
#45447=CARTESIAN_POINT('',(8.,4.,225.));
#45448=CARTESIAN_POINT('Origin',(0.,0.,225.));
#45449=CARTESIAN_POINT('',(-12.,-1.46957615897682E-15,225.));
#45450=CARTESIAN_POINT('Origin',(0.,0.,225.));
#45451=CARTESIAN_POINT('Origin',(0.,0.,225.));
#45452=CARTESIAN_POINT('Ctrl Pts',(25.8782388507408,2.51331533716111,9.85490600980488));
#45453=CARTESIAN_POINT('Ctrl Pts',(25.8254874142179,2.46522436200857,9.02187505333748));
#45454=CARTESIAN_POINT('Ctrl Pts',(25.719984541172,1.47678881906405,7.42156871988577));
#45455=CARTESIAN_POINT('Ctrl Pts',(25.5617302316032,-1.36226416922746,7.35610196821514));
#45456=CARTESIAN_POINT('Ctrl Pts',(25.4034759220345,-2.95646907341594,9.70130182803619));
#45457=CARTESIAN_POINT('Ctrl Pts',(25.2452216124657,-1.86324714060836,12.3157605506598));
#45458=CARTESIAN_POINT('Ctrl Pts',(25.0869673028969,0.926675464118667,12.8244356151764));
#45459=CARTESIAN_POINT('Ctrl Pts',(24.9287129933281,2.87272546418627,10.7625119609902));
#45460=CARTESIAN_POINT('Ctrl Pts',(24.7704586837593,2.20527713880316,8.00713739835836));
#45461=CARTESIAN_POINT('Ctrl Pts',(24.6122043741905,-0.468917913780222,
7.06486504705933));
#45462=CARTESIAN_POINT('Ctrl Pts',(24.4539500646218,-2.71635156248176,8.79333488723566));
#45463=CARTESIAN_POINT('Ctrl Pts',(24.295695755053,-2.49225709450323,11.6196872386657));
#45464=CARTESIAN_POINT('Ctrl Pts',(24.1374414454842,-0.000458301478133477,
12.9723291023825));
#45465=CARTESIAN_POINT('Ctrl Pts',(23.9791871359154,2.49174376617016,11.6204674958341));
#45466=CARTESIAN_POINT('Ctrl Pts',(23.8209328263466,2.71674214815707,8.794166840796));
#45467=CARTESIAN_POINT('Ctrl Pts',(23.6626785167778,0.469802408787728,7.06503722090339));
#45468=CARTESIAN_POINT('Ctrl Pts',(23.504424207209,-2.20460355977341,8.00640047512599));
#45469=CARTESIAN_POINT('Ctrl Pts',(23.3461698976402,-2.87306549282161,10.7617175021526));
#45470=CARTESIAN_POINT('Ctrl Pts',(23.1879155880715,-0.927355560621537,
12.8239564779555));
#45471=CARTESIAN_POINT('Ctrl Pts',(23.0296612785027,1.86214493867816,12.3167076110986));
#45472=CARTESIAN_POINT('Ctrl Pts',(22.8714069689339,2.9572999547598,9.70151157633143));
#45473=CARTESIAN_POINT('Ctrl Pts',(22.7131526593651,1.36163952175133,7.35790687334192));
#45474=CARTESIAN_POINT('Ctrl Pts',(22.5548983497963,-1.47296200852591,7.4183142853128));
#45475=CARTESIAN_POINT('Ctrl Pts',(22.3966440402275,-2.9673312917242,9.8277697035192));
#45476=CARTESIAN_POINT('Ctrl Pts',(22.2383897306587,-1.76175778279907,12.3939356232425));
#45477=CARTESIAN_POINT('Ctrl Pts',(22.08013542109,1.04682015196535,12.7818852987695));
#45478=CARTESIAN_POINT('Ctrl Pts',(21.9218811115212,2.90290770823478,10.6386275065772));
#45479=CARTESIAN_POINT('Ctrl Pts',(21.7636268019524,2.1176708058489,7.91428942327487));
#45480=CARTESIAN_POINT('Ctrl Pts',(21.6053724923836,-0.594411953138661,
7.08771692978175));
#45481=CARTESIAN_POINT('Ctrl Pts',(21.4471181828149,-2.76564567861122,8.91099943403972));
#45482=CARTESIAN_POINT('Ctrl Pts',(21.288863873246,-2.4204481889921,11.7251518241051));
#45483=CARTESIAN_POINT('Ctrl Pts',(21.1306095636773,0.127089037647067,12.9696071504951));
#45484=CARTESIAN_POINT('Ctrl Pts',(20.9723552541085,2.55898931782906,11.5120489155952));
#45485=CARTESIAN_POINT('Ctrl Pts',(20.8141009445397,2.66249277992261,8.67869365826803));
#45486=CARTESIAN_POINT('Ctrl Pts',(20.655846634971,0.34342273862104,7.04758080983749));
#45487=CARTESIAN_POINT('Ctrl Pts',(20.4975923254021,-2.28812395363916,8.10284238276193));
#45488=CARTESIAN_POINT('Ctrl Pts',(20.3393380158334,-2.8377313052884,10.8843072378062));
#45489=CARTESIAN_POINT('Ctrl Pts',(20.1810837062645,-0.805317506749925,
12.8611504618201));
#45490=CARTESIAN_POINT('Ctrl Pts',(20.0228293966958,1.95984601730847,12.2346636973589));
#45491=CARTESIAN_POINT('Ctrl Pts',(19.864575087127,2.94176675922726,9.57488050367255));
#45492=CARTESIAN_POINT('Ctrl Pts',(19.7063207775582,1.24700561195739,7.30190896083931));
#45493=CARTESIAN_POINT('Ctrl Pts',(19.5480664679894,-1.58239251044796,7.48390139407635));
#45494=CARTESIAN_POINT('Ctrl Pts',(19.3898121584206,-2.9719887311495,9.95526484857637));
#45495=CARTESIAN_POINT('Ctrl Pts',(19.2315578488518,-1.65740441592337,12.4673323355256));
#45496=CARTESIAN_POINT('Ctrl Pts',(19.0733035392831,1.16523432586418,12.7344007053979));
#45497=CARTESIAN_POINT('Ctrl Pts',(18.9150492297143,2.92763890499457,10.5134673249728));
#45498=CARTESIAN_POINT('Ctrl Pts',(18.7567949201455,2.02621637733479,7.82533555598277));
#45499=CARTESIAN_POINT('Ctrl Pts',(18.5985406105767,-0.718838608193511,
7.11590754183866));
#45500=CARTESIAN_POINT('Ctrl Pts',(18.4402863010079,-2.80983008655689,9.0306841915391));
#45501=CARTESIAN_POINT('Ctrl Pts',(18.2820319914391,-2.34418743313729,11.8274308551006));
#45502=CARTESIAN_POINT('Ctrl Pts',(18.1237776818704,0.254406117039017,12.9614178664055));
#45503=CARTESIAN_POINT('Ctrl Pts',(17.9655233723016,2.62151828146601,11.4008426577571));
#45504=CARTESIAN_POINT('Ctrl Pts',(17.8072690627328,2.603339197303,8.56565580294047));
#45505=CARTESIAN_POINT('Ctrl Pts',(17.649014753164,0.21640981742754,7.03556328406668));
#45506=CARTESIAN_POINT('Ctrl Pts',(17.4907604435952,-2.36742852442935,8.20277980381625));
#45507=CARTESIAN_POINT('Ctrl Pts',(17.3325061340264,-2.79716915088687,11.0052676226654));
#45508=CARTESIAN_POINT('Ctrl Pts',(17.1742518244576,-0.681795694559783,
12.8930732591368));
#45509=CARTESIAN_POINT('Ctrl Pts',(17.0159975148889,2.05393632079682,12.148502697686));
#45510=CARTESIAN_POINT('Ctrl Pts',(16.8577432053201,2.92081380029337,9.44903267259446));
#45511=CARTESIAN_POINT('Ctrl Pts',(16.6994888957513,1.13007426225585,7.25088188437829));
#45512=CARTESIAN_POINT('Ctrl Pts',(16.5412345861825,-1.68890767526181,7.55412405950459));
#45513=CARTESIAN_POINT('Ctrl Pts',(16.3829802766137,-2.97117070985973,10.0828424089713));
#45514=CARTESIAN_POINT('Ctrl Pts',(16.2247259670449,-1.54999751729083,12.5361833427899));
#45515=CARTESIAN_POINT('Ctrl Pts',(16.0664716574761,1.28150172162649,12.6818783695986));
#45516=CARTESIAN_POINT('Ctrl Pts',(15.9082173479074,2.9469763467695,10.3873611537488));
#45517=CARTESIAN_POINT('Ctrl Pts',(15.7499630383386,1.93102893513004,7.74038819627284));
#45518=CARTESIAN_POINT('Ctrl Pts',(15.5917087287698,-0.841940905955885,
7.14941168129618));
#45519=CARTESIAN_POINT('Ctrl Pts',(15.433454419201,-2.8488377850469,9.15215477453626));
#45520=CARTESIAN_POINT('Ctrl Pts',(15.2752001096322,-2.26360784764101,11.9263431064976));
#45521=CARTESIAN_POINT('Ctrl Pts',(15.1169458000635,0.381254489581041,12.9477725940152));
#45522=CARTESIAN_POINT('Ctrl Pts',(14.9586914904947,2.67921747312979,11.2870555479577));
#45523=CARTESIAN_POINT('Ctrl Pts',(14.8004371809259,2.53938933505717,8.455260521366));
#45524=CARTESIAN_POINT('Ctrl Pts',(14.6421828713571,0.0889981921416642,
7.02900730838193));
#45525=CARTESIAN_POINT('Ctrl Pts',(14.4839285617883,-2.44237144722633,8.30602834568397));
#45526=CARTESIAN_POINT('Ctrl Pts',(14.3256742522195,-2.75145361293339,11.1243759459044));
#45527=CARTESIAN_POINT('Ctrl Pts',(14.1674199426507,-0.55701777144916,12.9196659833176));
#45528=CARTESIAN_POINT('Ctrl Pts',(14.009165633082,2.14424254077798,12.0583833895003));
#45529=CARTESIAN_POINT('Ctrl Pts',(13.8509113235132,2.89447966024978,9.32419991990774));
#45530=CARTESIAN_POINT('Ctrl Pts',(13.6926570139444,1.01106091257489,7.20491966431815));
#45531=CARTESIAN_POINT('Ctrl Pts',(13.5344027043756,-1.79231126956862,7.62885290105586));
#45532=CARTESIAN_POINT('Ctrl Pts',(13.3761483948068,-2.96487873206638,10.2102673440928));
#45533=CARTESIAN_POINT('Ctrl Pts',(13.217894085238,-1.43973497022295,12.6003617954753));
#45534=CARTESIAN_POINT('Ctrl Pts',(13.0596397756693,1.39540813400357,12.6244150570019));
#45535=CARTESIAN_POINT('Ctrl Pts',(12.9013854661004,2.96088440668839,10.2605413250743));
#45536=CARTESIAN_POINT('Ctrl Pts',(12.7431311565317,1.83228384867635,7.65960384769567));
#45537=CARTESIAN_POINT('Ctrl Pts',(12.5848768469629,-0.963492048187264,
7.18816762146178));
#45538=CARTESIAN_POINT('Ctrl Pts',(12.4266225373941,-2.88259690791579,9.27518739095129));
#45539=CARTESIAN_POINT('Ctrl Pts',(12.2683682278253,-2.17885788889992,12.0217063465763));
#45540=CARTESIAN_POINT('Ctrl Pts',(12.1101139182565,0.507400455370921,12.9286964728651));
#45541=CARTESIAN_POINT('Ctrl Pts',(11.9518596086877,2.73198059023493,11.170897222515));
#45542=CARTESIAN_POINT('Ctrl Pts',(11.793605299119,2.47076101180668,8.34771120128963));
#45543=CARTESIAN_POINT('Ctrl Pts',(11.6353509895502,-0.0385773998656385,
7.0279249607546));
#45544=CARTESIAN_POINT('Ctrl Pts',(11.4770966799814,-2.51281464985175,8.41239778862548));
#45545=CARTESIAN_POINT('Ctrl Pts',(11.3188423704126,-2.70066891686761,11.2414127657423));
#45546=CARTESIAN_POINT('Ctrl Pts',(11.1605880608438,-0.43121362073721,12.9408796444537));
#45547=CARTESIAN_POINT('Ctrl Pts',(11.0023337512751,2.2305982968671,11.9644717982181));
#45548=CARTESIAN_POINT('Ctrl Pts',(10.8440794417063,2.862812863889,9.20061224460173));
#45549=CARTESIAN_POINT('Ctrl Pts',(10.6858251321375,0.890184812731906,7.16410695535464));
#45550=CARTESIAN_POINT('Ctrl Pts',(10.5275708225687,-1.89241275771817,7.70795028797535));
#45551=CARTESIAN_POINT('Ctrl Pts',(10.3693165129999,-2.95312444633263,10.33730480233));
#45552=CARTESIAN_POINT('Ctrl Pts',(10.2110622034311,-1.32681980887658,12.659749626168));
#45553=CARTESIAN_POINT('Ctrl Pts',(10.0528078938623,1.50674349723582,12.5621163039333));
#45554=CARTESIAN_POINT('Ctrl Pts',(9.89455358429355,2.96933786459887,10.1332421248879));
#45555=CARTESIAN_POINT('Ctrl Pts',(9.73629927472478,1.73016226470662,7.58313011413639));
#45556=CARTESIAN_POINT('Ctrl Pts',(9.57804496515598,-1.08326659812887,7.23210632814751));
#45557=CARTESIAN_POINT('Ctrl Pts',(9.4197906555872,-2.9110481400647,9.39955081052956));
#45558=CARTESIAN_POINT('Ctrl Pts',(9.26153634601842,-2.09008814807197,12.1133536640817));
#45559=CARTESIAN_POINT('Ctrl Pts',(9.10328203644963,0.63260092362554,12.9042077365071));
#45560=CARTESIAN_POINT('Ctrl Pts',(8.94502772688085,2.77973100053036,11.0526142534321));
#45561=CARTESIAN_POINT('Ctrl Pts',(8.78677341731206,2.39754104106069,8.24314327152743));
#45562=CARTESIAN_POINT('Ctrl Pts',(8.62851910774328,-0.166005611993985,
7.03243901157466));
#45563=CARTESIAN_POINT('Ctrl Pts',(8.47026479817449,-2.57877530773441,8.52145954661513));
#45564=CARTESIAN_POINT('Ctrl Pts',(8.31201048860571,-2.64462552602106,11.3566107260726));
#45565=CARTESIAN_POINT('Ctrl Pts',(8.15375617903693,-0.305161145104408,
12.9558089680353));
#45566=CARTESIAN_POINT('Ctrl Pts',(7.99550186946814,2.31390515511262,11.868636776471));
#45567=CARTESIAN_POINT('Ctrl Pts',(7.83724755989935,2.82374457369778,9.07497045187927));
#45568=CARTESIAN_POINT('Ctrl Pts',(7.7317446868535,1.45630799602658,7.78342006978472));
#45569=CARTESIAN_POINT('Ctrl Pts',(7.67899325033057,0.650199997975098,7.56791319796493));
#45570=CARTESIAN_POINT('Ctrl Pts',(25.9852411006306,2.69834060395509,9.84422447937807));
#45571=CARTESIAN_POINT('Ctrl Pts',(25.9324896641077,2.64670926704356,8.94986744389102));
#45572=CARTESIAN_POINT('Ctrl Pts',(25.8269867910618,1.58550706910041,7.23174974712926));
#45573=CARTESIAN_POINT('Ctrl Pts',(25.668732481493,-1.46255134275814,7.1614634636574));
#45574=CARTESIAN_POINT('Ctrl Pts',(25.5104781719243,-3.17411843519274,9.67931226383733));
#45575=CARTESIAN_POINT('Ctrl Pts',(25.3522238623555,-2.0004156821745,12.4862422277425));
#45576=CARTESIAN_POINT('Ctrl Pts',(25.1939695527867,0.994895465184538,13.032364936863));
#45577=CARTESIAN_POINT('Ctrl Pts',(25.0357152432179,3.08420978832894,10.8186465720873));
#45578=CARTESIAN_POINT('Ctrl Pts',(24.8774609336491,2.36762524726719,7.86042682483797));
#45579=CARTESIAN_POINT('Ctrl Pts',(24.7192066240803,-0.503438716171723,
6.84878626071905));
#45580=CARTESIAN_POINT('Ctrl Pts',(24.5609523145115,-2.91632395158999,8.70450260617681));
#45581=CARTESIAN_POINT('Ctrl Pts',(24.4026980049428,-2.67573209543587,11.738925385597));
#45582=CARTESIAN_POINT('Ctrl Pts',(24.244443695374,-0.00049204071968808,
13.1911460478872));
#45583=CARTESIAN_POINT('Ctrl Pts',(24.0861893858052,2.67518097689384,11.7397630837433));
#45584=CARTESIAN_POINT('Ctrl Pts',(23.9279350762364,2.91674329140439,8.70539580650041));
#45585=CARTESIAN_POINT('Ctrl Pts',(23.7696807666676,0.504388325939132,6.84897110965841));
#45586=CARTESIAN_POINT('Ctrl Pts',(23.6114264570989,-2.36690208069152,7.85963565078572));
#45587=CARTESIAN_POINT('Ctrl Pts',(23.45317214753,-3.08457484919484,10.8177936267731));
#45588=CARTESIAN_POINT('Ctrl Pts',(23.2949178379613,-0.995625629036708,
13.0318505265147));
#45589=CARTESIAN_POINT('Ctrl Pts',(23.1366635283925,1.99923233833457,12.4872590088835));
#45590=CARTESIAN_POINT('Ctrl Pts',(22.9784092188237,3.17501048436542,9.67953745338411));
#45591=CARTESIAN_POINT('Ctrl Pts',(22.8201549092549,1.46188070997956,7.16340124230294));
#45592=CARTESIAN_POINT('Ctrl Pts',(22.6619005996861,-1.5813985363962,7.2282557275682));
#45593=CARTESIAN_POINT('Ctrl Pts',(22.5036462901173,-3.18578030836752,9.81509045229863));
#45594=CARTESIAN_POINT('Ctrl Pts',(22.3453919805486,-1.89145488008292,12.5701723933879));
#45595=CARTESIAN_POINT('Ctrl Pts',(22.1871376709798,1.12388496553606,12.986682150953));
#45596=CARTESIAN_POINT('Ctrl Pts',(22.028883361411,3.11661398903962,10.6856419910071));
#45597=CARTESIAN_POINT('Ctrl Pts',(21.8706290518422,2.27356951065551,7.76074356684863));
#45598=CARTESIAN_POINT('Ctrl Pts',(21.7123747422734,-0.638171376633541,
6.87332045351015));
#45599=CARTESIAN_POINT('Ctrl Pts',(21.5541204327046,-2.96924700231964,8.83082938244435));
#45600=CARTESIAN_POINT('Ctrl Pts',(21.3958661231359,-2.59863676139588,11.8521540636552));
#45601=CARTESIAN_POINT('Ctrl Pts',(21.2376118135671,0.136445079346075,13.188223711326));
#45602=CARTESIAN_POINT('Ctrl Pts',(21.0793575039983,2.74737701206447,11.6233629436748));
#45603=CARTESIAN_POINT('Ctrl Pts',(20.9211031944295,2.85850019278417,8.58142171838018));
#45604=CARTESIAN_POINT('Ctrl Pts',(20.7628488848607,0.36870483629377,6.83022959239551));
#45605=CARTESIAN_POINT('Ctrl Pts',(20.6045945752919,-2.4565710795211,7.96317741948034));
#45606=CARTESIAN_POINT('Ctrl Pts',(20.4463402657232,-3.0466394291865,10.9494081744789));
#45607=CARTESIAN_POINT('Ctrl Pts',(20.2880859561544,-0.86460337682645,13.0717826573543));
#45608=CARTESIAN_POINT('Ctrl Pts',(20.1298316465856,2.10412597568299,12.3991751857047));
#45609=CARTESIAN_POINT('Ctrl Pts',(19.9715773370168,3.15833376593105,9.54358405349603));
#45610=CARTESIAN_POINT('Ctrl Pts',(19.813323027448,1.33880768017961,7.10328087506992));
#45611=CARTESIAN_POINT('Ctrl Pts',(19.6550687178792,-1.69888509380567,7.29867122858234));
#45612=CARTESIAN_POINT('Ctrl Pts',(19.4968144083105,-3.19078061920234,9.95197153587308));
#45613=CARTESIAN_POINT('Ctrl Pts',(19.3385600987416,-1.77941922628463,12.6489724253703));
#45614=CARTESIAN_POINT('Ctrl Pts',(19.1803057891729,1.2510165549513,12.9357018364408));
#45615=CARTESIAN_POINT('Ctrl Pts',(19.0220514796041,3.14316584722257,10.5512677662419));
#45616=CARTESIAN_POINT('Ctrl Pts',(18.8637971700353,2.17538238935706,7.66524109310643));
#45617=CARTESIAN_POINT('Ctrl Pts',(18.7055428604665,-0.77175807408634,6.90358640225075));
#45618=CARTESIAN_POINT('Ctrl Pts',(18.5472885508978,-3.01668417833122,8.95932509329292));
#45619=CARTESIAN_POINT('Ctrl Pts',(18.389034241329,-2.51676184066121,11.9619626730994));
#45620=CARTESIAN_POINT('Ctrl Pts',(18.2307799317602,0.27313498841587,13.1794315484606));
#45621=CARTESIAN_POINT('Ctrl Pts',(18.0725256221914,2.81450923340181,11.5039699027373));
#45622=CARTESIAN_POINT('Ctrl Pts',(17.9142713126226,2.79499184128849,8.46006224139594));
#45623=CARTESIAN_POINT('Ctrl Pts',(17.7560170030538,0.232341476942896,6.81732736032501));
#45624=CARTESIAN_POINT('Ctrl Pts',(17.597762693485,-2.54171389478125,8.07047203432559));
#45625=CARTESIAN_POINT('Ctrl Pts',(17.4395083839162,-3.00309116980684,11.0792734218315));
#45626=CARTESIAN_POINT('Ctrl Pts',(17.2812540743475,-0.731988134966967,
13.1060555473963));
#45627=CARTESIAN_POINT('Ctrl Pts',(17.1229997647787,2.20514301981873,12.3066711849304));
#45628=CARTESIAN_POINT('Ctrl Pts',(16.9647454552099,3.13583829191377,9.40847155587319));
#45629=CARTESIAN_POINT('Ctrl Pts',(16.8064911456411,1.21326807752421,7.04849728692239));
#45630=CARTESIAN_POINT('Ctrl Pts',(16.6482368360723,-1.81324169279846,7.37406354670546));
#45631=CARTESIAN_POINT('Ctrl Pts',(16.4899825265035,-3.1899023768153,10.0889411020383));
#45632=CARTESIAN_POINT('Ctrl Pts',(16.3317282169347,-1.66410524580638,12.7228921065888));
#45633=CARTESIAN_POINT('Ctrl Pts',(16.173473907366,1.37584332470155,12.8793129109421));
#45634=CARTESIAN_POINT('Ctrl Pts',(16.0152195977972,3.16392687292691,10.4158779099864));
#45635=CARTESIAN_POINT('Ctrl Pts',(15.8569652882284,2.07318743733889,7.57404007805077));
#45636=CARTESIAN_POINT('Ctrl Pts',(15.6987109786596,-0.90392291770186,6.93955704969084));
#45637=CARTESIAN_POINT('Ctrl Pts',(15.5404566690908,-3.05856354585273,9.08973809855375));
#45638=CARTESIAN_POINT('Ctrl Pts',(15.3822023595221,-2.43025014665305,12.06815664734));
#45639=CARTESIAN_POINT('Ctrl Pts',(15.2239480499532,0.409321685371451,13.1647817383081));
#45640=CARTESIAN_POINT('Ctrl Pts',(15.0656937403845,2.87645612457767,11.38180601266));
#45641=CARTESIAN_POINT('Ctrl Pts',(14.9074394308157,2.72633411761815,8.34153987917857));
#45642=CARTESIAN_POINT('Ctrl Pts',(14.7491851212469,0.0955500616988636,
6.81028874677455));
#45643=CARTESIAN_POINT('Ctrl Pts',(14.5909308116781,-2.62217396621445,8.18132152810044));
#45644=CARTESIAN_POINT('Ctrl Pts',(14.4326765021093,-2.95401014504738,11.2071502624781));
#45645=CARTESIAN_POINT('Ctrl Pts',(14.2744221925406,-0.598024309804106,
13.1346059749396));
#45646=CARTESIAN_POINT('Ctrl Pts',(14.1161678829718,2.30209740376012,12.2099174728584));
#45647=CARTESIAN_POINT('Ctrl Pts',(13.957913573403,3.10756548495669,9.27444886469009));
#45648=CARTESIAN_POINT('Ctrl Pts',(13.7996592638342,1.08549320219973,6.99915141981115));
#45649=CARTESIAN_POINT('Ctrl Pts',(13.6414049542654,-1.92425765366397,7.45429377665825));
#45650=CARTESIAN_POINT('Ctrl Pts',(13.4831506446966,-3.18314719615494,10.2257468069615));
#45651=CARTESIAN_POINT('Ctrl Pts',(13.3248963351278,-1.54572538974549,12.7917952490713));
#45652=CARTESIAN_POINT('Ctrl Pts',(13.1666420255591,1.4981353001745,12.8176192637802));
#45653=CARTESIAN_POINT('Ctrl Pts',(13.0083877159903,3.17885881650219,10.2797218582409));
#45654=CARTESIAN_POINT('Ctrl Pts',(12.8501334064215,1.96717293439155,7.48730854671172));
#45655=CARTESIAN_POINT('Ctrl Pts',(12.6918790968527,-1.03442241280721,6.9811661249418));
#45656=CARTESIAN_POINT('Ctrl Pts',(12.5336247872839,-3.09480794807483,9.22182813101998));
#45657=CARTESIAN_POINT('Ctrl Pts',(12.3753704777151,-2.33926106483218,12.1705403391213));
#45658=CARTESIAN_POINT('Ctrl Pts',(12.2171161681464,0.54475426578949,13.1443012711322));
#45659=CARTESIAN_POINT('Ctrl Pts',(12.0588618585775,2.9331035572221,11.257096342769));
#45660=CARTESIAN_POINT('Ctrl Pts',(11.9006075490088,2.65265351396683,8.22607299247362));
#45661=CARTESIAN_POINT('Ctrl Pts',(11.74235323944,-0.0414173911698831,6.80912671887172));
#45662=CARTESIAN_POINT('Ctrl Pts',(11.5840989298712,-2.69780305704375,8.29552167746703));
#45663=CARTESIAN_POINT('Ctrl Pts',(11.4258446203024,-2.89948678085681,11.3328030997711));
#45664=CARTESIAN_POINT('Ctrl Pts',(11.2675903107337,-0.462958708208892,
13.1573813435356));
#45665=CARTESIAN_POINT('Ctrl Pts',(11.1093360011649,2.39481049852988,12.1090922973653));
#45666=CARTESIAN_POINT('Ctrl Pts',(10.9510816915961,3.07356744215081,9.14176291100341));
#45667=CARTESIAN_POINT('Ctrl Pts',(10.7928273820273,0.955718444758249,6.95533416054196));
#45668=CARTESIAN_POINT('Ctrl Pts',(10.6345730724585,-2.03172841389709,7.53921415558398));
#45669=CARTESIAN_POINT('Ctrl Pts',(10.4763187628897,-3.17052758332845,10.3621365097244));
#45670=CARTESIAN_POINT('Ctrl Pts',(10.3180644533209,-1.42449763922883,12.8555550935164));
#45671=CARTESIAN_POINT('Ctrl Pts',(10.1598101437521,1.61766695098797,12.7507342006546));
#45672=CARTESIAN_POINT('Ctrl Pts',(10.0015558341834,3.18793460113869,10.1430511446082));
#45673=CARTESIAN_POINT('Ctrl Pts',(9.84330152461458,1.85753336290945,7.4052049692784));
#45674=CARTESIAN_POINT('Ctrl Pts',(9.6850472150458,-1.16301452643865,7.02833951165627));
#45675=CARTESIAN_POINT('Ctrl Pts',(9.52679290547701,-3.12535370323928,9.35534693772645));
#45676=CARTESIAN_POINT('Ctrl Pts',(9.36853859590823,-2.2439562725775,12.2689345495142));
#45677=CARTESIAN_POINT('Ctrl Pts',(9.21028428633944,0.679171743027831,13.1180097228028));
#45678=CARTESIAN_POINT('Ctrl Pts',(9.05202997677066,2.9843692575704,11.1301056172068));
#45679=CARTESIAN_POINT('Ctrl Pts',(8.89377566720187,2.57404323488125,8.11380698009667));
#45680=CARTESIAN_POINT('Ctrl Pts',(8.73552135763309,-0.178226614346673,
6.81397308511794));
#45681=CARTESIAN_POINT('Ctrl Pts',(8.57726704806431,-2.76861960711876,8.41261234475057));
#45682=CARTESIAN_POINT('Ctrl Pts',(8.41901273849552,-2.83931758725479,11.456481704384));
#45683=CARTESIAN_POINT('Ctrl Pts',(8.26075842892673,-0.327626500506996,
13.1734097341694));
#45684=CARTESIAN_POINT('Ctrl Pts',(8.10250411935795,2.48425024167238,12.0062020922894));
#45685=CARTESIAN_POINT('Ctrl Pts',(7.94424980978916,3.03162302228778,9.00687161986933));
#45686=CARTESIAN_POINT('Ctrl Pts',(7.83874693674331,1.56351848868342,7.62023987234021));
#45687=CARTESIAN_POINT('Ctrl Pts',(7.78599550022038,0.698066426161017,7.38886781406139));
#45688=CARTESIAN_POINT('Ctrl Pts',(26.0922433505204,2.88336587074908,9.83354294895125));
#45689=CARTESIAN_POINT('Ctrl Pts',(26.0394919139975,2.82819417207855,8.87785983444456));
#45690=CARTESIAN_POINT('Ctrl Pts',(25.9339890409517,1.69422531913677,7.04193077437275));
#45691=CARTESIAN_POINT('Ctrl Pts',(25.7757347313828,-1.56283851628882,6.96682495909965));
#45692=CARTESIAN_POINT('Ctrl Pts',(25.6174804218141,-3.39176779696954,9.65732269963848));
#45693=CARTESIAN_POINT('Ctrl Pts',(25.4592261122453,-2.13758422374064,12.6567239048252));
#45694=CARTESIAN_POINT('Ctrl Pts',(25.3009718026765,1.06311546625041,13.2402942585496));
#45695=CARTESIAN_POINT('Ctrl Pts',(25.1427174931077,3.29569411247162,10.8747811831844));
#45696=CARTESIAN_POINT('Ctrl Pts',(24.9844631835389,2.52997335573122,7.71371625131757));
#45697=CARTESIAN_POINT('Ctrl Pts',(24.8262088739702,-0.537959518563222,
6.63270747437876));
#45698=CARTESIAN_POINT('Ctrl Pts',(24.6679545644013,-3.11629634069821,8.61567032511795));
#45699=CARTESIAN_POINT('Ctrl Pts',(24.5097002548326,-2.85920709636852,11.8581635325282));
#45700=CARTESIAN_POINT('Ctrl Pts',(24.3514459452638,-0.000525779961243345,
13.409962993392));
#45701=CARTESIAN_POINT('Ctrl Pts',(24.193191635695,2.85861818761752,11.8590586716524));
#45702=CARTESIAN_POINT('Ctrl Pts',(24.0349373261262,3.1167444346517,8.61662477220482));
#45703=CARTESIAN_POINT('Ctrl Pts',(23.8766830165574,0.538974243090536,6.63290499841343));
#45704=CARTESIAN_POINT('Ctrl Pts',(23.7184287069887,-2.52920060160962,7.71287082644543));
#45705=CARTESIAN_POINT('Ctrl Pts',(23.5601743974198,-3.29608420556807,10.8738697513937));
#45706=CARTESIAN_POINT('Ctrl Pts',(23.4019200878511,-1.06389569745188,13.2397445750738));
#45707=CARTESIAN_POINT('Ctrl Pts',(23.2436657782823,2.13631973799098,12.6578104066685));
#45708=CARTESIAN_POINT('Ctrl Pts',(23.0854114687135,3.39272101397104,9.65756333043674));
#45709=CARTESIAN_POINT('Ctrl Pts',(22.9271571591447,1.5621218982078,6.96889561126398));
#45710=CARTESIAN_POINT('Ctrl Pts',(22.768902849576,-1.6898350642665,7.03819716982359));
#45711=CARTESIAN_POINT('Ctrl Pts',(22.6106485400071,-3.40422932501084,9.80241120107808));
#45712=CARTESIAN_POINT('Ctrl Pts',(22.4523942304384,-2.02115197736677,12.7464091635333));
#45713=CARTESIAN_POINT('Ctrl Pts',(22.2941399208696,1.20094977910676,13.1914790031365));
#45714=CARTESIAN_POINT('Ctrl Pts',(22.1358856113008,3.33032026984446,10.732656475437));
#45715=CARTESIAN_POINT('Ctrl Pts',(21.977631301732,2.42946821546214,7.6071977104224));
#45716=CARTESIAN_POINT('Ctrl Pts',(21.8193769921633,-0.681930800128424,
6.65892397723854));
#45717=CARTESIAN_POINT('Ctrl Pts',(21.6611226825944,-3.17284832602806,8.750659330849));
#45718=CARTESIAN_POINT('Ctrl Pts',(21.5028683730257,-2.77682533379967,11.9791563032054));
#45719=CARTESIAN_POINT('Ctrl Pts',(21.3446140634568,0.145801121045086,13.4068402721569));
#45720=CARTESIAN_POINT('Ctrl Pts',(21.1863597538881,2.93576470629988,11.7346769717544));
#45721=CARTESIAN_POINT('Ctrl Pts',(21.0281054443193,3.05450760564573,8.48414977849232));
#45722=CARTESIAN_POINT('Ctrl Pts',(20.8698511347506,0.393986933966499,6.61287837495358));
#45723=CARTESIAN_POINT('Ctrl Pts',(20.7115968251817,-2.62501820540304,7.82351245619871));
#45724=CARTESIAN_POINT('Ctrl Pts',(20.553342515613,-3.25554755308459,11.0145091111515));
#45725=CARTESIAN_POINT('Ctrl Pts',(20.3950882060442,-0.923889246902975,
13.2824148528885));
#45726=CARTESIAN_POINT('Ctrl Pts',(20.2368338964754,2.2484059340575,12.5636866740505));
#45727=CARTESIAN_POINT('Ctrl Pts',(20.0785795869066,3.37490077263483,9.51228760331953));
#45728=CARTESIAN_POINT('Ctrl Pts',(19.9203252773378,1.43060974840183,6.90465278930053));
#45729=CARTESIAN_POINT('Ctrl Pts',(19.762070967769,-1.81537767716337,7.11344106308832));
#45730=CARTESIAN_POINT('Ctrl Pts',(19.6038166582003,-3.40957250725519,9.9486782231698));
#45731=CARTESIAN_POINT('Ctrl Pts',(19.4455623486315,-1.90143403664589,12.830612515215));
#45732=CARTESIAN_POINT('Ctrl Pts',(19.2873080390627,1.33679878403842,13.1370029674836));
#45733=CARTESIAN_POINT('Ctrl Pts',(19.1290537294939,3.35869278945057,10.589068207511));
#45734=CARTESIAN_POINT('Ctrl Pts',(18.9707994199251,2.32454840137932,7.50514663023009));
#45735=CARTESIAN_POINT('Ctrl Pts',(18.8125451103563,-0.824677539979167,
6.69126526266284));
#45736=CARTESIAN_POINT('Ctrl Pts',(18.6542908007876,-3.22353827010556,8.88796599504674));
#45737=CARTESIAN_POINT('Ctrl Pts',(18.4960364912188,-2.68933624818511,12.0964944910982));
#45738=CARTESIAN_POINT('Ctrl Pts',(18.33778218165,0.291863859792721,13.3974452305158));
#45739=CARTESIAN_POINT('Ctrl Pts',(18.1795278720812,3.00750018533761,11.6070971477175));
#45740=CARTESIAN_POINT('Ctrl Pts',(18.0212735625124,2.98664448527398,8.3544686798514));
#45741=CARTESIAN_POINT('Ctrl Pts',(17.8630192529436,0.248273136458253,6.59909143658335));
#45742=CARTESIAN_POINT('Ctrl Pts',(17.7047649433748,-2.71599926513316,7.93816426483493));
#45743=CARTESIAN_POINT('Ctrl Pts',(17.5465106338061,-3.20901318872681,11.1532792209976));
#45744=CARTESIAN_POINT('Ctrl Pts',(17.3882563242373,-0.78218057537415,13.3190378356558));
#45745=CARTESIAN_POINT('Ctrl Pts',(17.2300020146685,2.35634971884065,12.4648396721749));
#45746=CARTESIAN_POINT('Ctrl Pts',(17.0717477050997,3.35086278353417,9.36791043915191));
#45747=CARTESIAN_POINT('Ctrl Pts',(16.9134933955309,1.29646189279257,6.84611268946649));
#45748=CARTESIAN_POINT('Ctrl Pts',(16.7552390859622,-1.93757571033511,7.19400303390634));
#45749=CARTESIAN_POINT('Ctrl Pts',(16.5969847763933,-3.40863404377088,10.0950397951052));
#45750=CARTESIAN_POINT('Ctrl Pts',(16.4387304668246,-1.77821297432193,12.9096008703877));
#45751=CARTESIAN_POINT('Ctrl Pts',(16.2804761572558,1.4701849277766,13.0767474522856));
#45752=CARTESIAN_POINT('Ctrl Pts',(16.122221847687,3.38087739908433,10.444394666224));
#45753=CARTESIAN_POINT('Ctrl Pts',(15.9639675381182,2.21534593954773,7.40769195982868));
#45754=CARTESIAN_POINT('Ctrl Pts',(15.8057132285494,-0.965904929447833,
6.72970241808549));
#45755=CARTESIAN_POINT('Ctrl Pts',(15.6474589189806,-3.26828930665857,9.02732142257126));
#45756=CARTESIAN_POINT('Ctrl Pts',(15.4892046094119,-2.59689244566508,12.2099701881825));
#45757=CARTESIAN_POINT('Ctrl Pts',(15.3309502998431,0.437388881161856,13.381790882601));
#45758=CARTESIAN_POINT('Ctrl Pts',(15.1726959902743,3.07369477602556,11.4765564773624));
#45759=CARTESIAN_POINT('Ctrl Pts',(15.0144416807055,2.91327890017913,8.22781923699113));
#45760=CARTESIAN_POINT('Ctrl Pts',(14.8561873711367,0.102101931256069,6.59157018516719));
#45761=CARTESIAN_POINT('Ctrl Pts',(14.6979330615679,-2.80197648520258,8.0566147105169));
#45762=CARTESIAN_POINT('Ctrl Pts',(14.5396787519991,-3.15656667716138,11.2899245790518));
#45763=CARTESIAN_POINT('Ctrl Pts',(14.3814244424304,-0.639030848159055,
13.3495459665615));
#45764=CARTESIAN_POINT('Ctrl Pts',(14.2231701328616,2.45995226674225,12.3614515562165));
#45765=CARTESIAN_POINT('Ctrl Pts',(14.0649158232928,3.32065130966359,9.22469780947245));
#45766=CARTESIAN_POINT('Ctrl Pts',(13.906661513724,1.15992549182458,6.79338317530414));
#45767=CARTESIAN_POINT('Ctrl Pts',(13.7484072041552,-2.05620403775932,7.27973465226065));
#45768=CARTESIAN_POINT('Ctrl Pts',(13.5901528945864,-3.40141566024351,10.2412262698301));
#45769=CARTESIAN_POINT('Ctrl Pts',(13.4318985850176,-1.65171580926802,12.9832287026674));
#45770=CARTESIAN_POINT('Ctrl Pts',(13.2736442754489,1.60086246634544,13.0108234705585));
#45771=CARTESIAN_POINT('Ctrl Pts',(13.1153899658801,3.396833226316,10.2989023914076));
#45772=CARTESIAN_POINT('Ctrl Pts',(12.9571356563113,2.10206202010675,7.31501324572778));
#45773=CARTESIAN_POINT('Ctrl Pts',(12.7988813467425,-1.10535277742715,6.7741646284218));
#45774=CARTESIAN_POINT('Ctrl Pts',(12.6406270371737,-3.30701898823388,9.16846887108869));
#45775=CARTESIAN_POINT('Ctrl Pts',(12.482372727605,-2.49966424076443,12.3193743316664));
#45776=CARTESIAN_POINT('Ctrl Pts',(12.3241184180362,0.582108076208057,13.3599060693994));
#45777=CARTESIAN_POINT('Ctrl Pts',(12.1658641084674,3.13422652420927,11.3432954630231));
#45778=CARTESIAN_POINT('Ctrl Pts',(12.0076097988986,2.83454601612698,8.1044347836576));
#45779=CARTESIAN_POINT('Ctrl Pts',(11.8493554893298,-0.0442573824741247,
6.59032847698884));
#45780=CARTESIAN_POINT('Ctrl Pts',(11.691101179761,-2.88279146423575,8.17864556630858));
#45781=CARTESIAN_POINT('Ctrl Pts',(11.5328468701922,-3.098304644846,11.4241934337999));
#45782=CARTESIAN_POINT('Ctrl Pts',(11.3745925606235,-0.494703795680576,
13.3738830426176));
#45783=CARTESIAN_POINT('Ctrl Pts',(11.2163382510547,2.55902270019265,12.2537127965125));
#45784=CARTESIAN_POINT('Ctrl Pts',(11.0580839414859,3.28432202041261,9.08291357740508));
#45785=CARTESIAN_POINT('Ctrl Pts',(10.8998296319171,1.02125207678459,6.74656136572925));
#45786=CARTESIAN_POINT('Ctrl Pts',(10.7415753223483,-2.17104407007601,7.37047802319264));
#45787=CARTESIAN_POINT('Ctrl Pts',(10.5833210127795,-3.38793072032428,10.3869682171186));
#45788=CARTESIAN_POINT('Ctrl Pts',(10.4250667032107,-1.52217546958108,13.0513605608649));
#45789=CARTESIAN_POINT('Ctrl Pts',(10.266812393642,1.72859040474012,12.9393520973757));
#45790=CARTESIAN_POINT('Ctrl Pts',(10.1085580840732,3.40653133767851,10.1528601643285));
#45791=CARTESIAN_POINT('Ctrl Pts',(9.95030377450439,1.98490446111228,7.22727982442037));
#45792=CARTESIAN_POINT('Ctrl Pts',(9.79204946493561,-1.24276245474844,6.82457269516505));
#45793=CARTESIAN_POINT('Ctrl Pts',(9.63379515536682,-3.33965926641385,9.31114306492331));
#45794=CARTESIAN_POINT('Ctrl Pts',(9.47554084579804,-2.39782439708303,12.4245154349468));
#45795=CARTESIAN_POINT('Ctrl Pts',(9.31728653622925,0.725742562430119,13.3318117090984));
#45796=CARTESIAN_POINT('Ctrl Pts',(9.15903222666047,3.18900751461044,11.2075969809815));
#45797=CARTESIAN_POINT('Ctrl Pts',(9.00077791709168,2.7505454287018,7.98447068866592));
#45798=CARTESIAN_POINT('Ctrl Pts',(8.8425236075229,-0.190447616699357,6.5955071586612));
#45799=CARTESIAN_POINT('Ctrl Pts',(8.68426929795412,-2.95846390650311,8.30376514288603));
#45800=CARTESIAN_POINT('Ctrl Pts',(8.52601498838534,-3.03400964848852,11.5563526826953));
#45801=CARTESIAN_POINT('Ctrl Pts',(8.36776067881654,-0.350091855909584,
13.3910105003035));
#45802=CARTESIAN_POINT('Ctrl Pts',(8.20950636924776,2.65459532823215,12.1437674081077));
#45803=CARTESIAN_POINT('Ctrl Pts',(8.05125205967898,3.23950147087779,8.93877278785939));
#45804=CARTESIAN_POINT('Ctrl Pts',(7.94574918663312,1.67072898134026,7.45705967489569));
#45805=CARTESIAN_POINT('Ctrl Pts',(7.89299775011019,0.745932854346936,7.20982243015784));
#45806=CARTESIAN_POINT('Ctrl Pts',(26.1992456004102,3.06839113754307,9.82286141852444));
#45807=CARTESIAN_POINT('Ctrl Pts',(26.1464941638873,3.00967907711354,8.80585222499811));
#45808=CARTESIAN_POINT('Ctrl Pts',(26.0409912908414,1.80294356917313,6.85211180161624));
#45809=CARTESIAN_POINT('Ctrl Pts',(25.8827369812727,-1.66312568981951,6.77218645454191));
#45810=CARTESIAN_POINT('Ctrl Pts',(25.7244826717039,-3.60941715874633,9.63533313543961));
#45811=CARTESIAN_POINT('Ctrl Pts',(25.5662283621351,-2.27475276530677,12.8272055819078));
#45812=CARTESIAN_POINT('Ctrl Pts',(25.4079740525663,1.13133546731627,13.4482235802362));
#45813=CARTESIAN_POINT('Ctrl Pts',(25.2497197429975,3.5071784366143,10.9309157942814));
#45814=CARTESIAN_POINT('Ctrl Pts',(25.0914654334287,2.69232146419524,7.56700567779718));
#45815=CARTESIAN_POINT('Ctrl Pts',(24.93321112386,-0.572480320954722,6.41662868803847));
#45816=CARTESIAN_POINT('Ctrl Pts',(24.7749568142912,-3.31626872980643,8.5268380440591));
#45817=CARTESIAN_POINT('Ctrl Pts',(24.6167025047224,-3.04268209730116,11.9774016794594));
#45818=CARTESIAN_POINT('Ctrl Pts',(24.4584481951536,-0.000559519202797285,
13.6287799388967));
#45819=CARTESIAN_POINT('Ctrl Pts',(24.3001938855848,3.04205539834121,11.9783542595615));
#45820=CARTESIAN_POINT('Ctrl Pts',(24.141939576016,3.31674557789901,8.52785373790922));
#45821=CARTESIAN_POINT('Ctrl Pts',(23.9836852664473,0.573560160241939,6.41683888716847));
#45822=CARTESIAN_POINT('Ctrl Pts',(23.8254309568785,-2.69149912252773,7.56610600210514));
#45823=CARTESIAN_POINT('Ctrl Pts',(23.6671766473097,-3.5075935619413,10.9299458760143));
#45824=CARTESIAN_POINT('Ctrl Pts',(23.5089223377409,-1.13216576586705,13.447638623633));
#45825=CARTESIAN_POINT('Ctrl Pts',(23.3506680281721,2.27340713764739,12.8283618044535));
#45826=CARTESIAN_POINT('Ctrl Pts',(23.1924137186033,3.61043154357666,9.63558920748943));
#45827=CARTESIAN_POINT('Ctrl Pts',(23.0341594090345,1.66236308643603,6.77438998022499));
#45828=CARTESIAN_POINT('Ctrl Pts',(22.8759050994658,-1.79827159213679,6.848138612079));
#45829=CARTESIAN_POINT('Ctrl Pts',(22.7176507898969,-3.62267834165416,9.7897319498575));
#45830=CARTESIAN_POINT('Ctrl Pts',(22.5593964803283,-2.15084907465062,12.9226459336786));
#45831=CARTESIAN_POINT('Ctrl Pts',(22.4011421707594,1.27801459267746,13.39627585532));
#45832=CARTESIAN_POINT('Ctrl Pts',(22.2428878611907,3.5440265506493,10.7796709598669));
#45833=CARTESIAN_POINT('Ctrl Pts',(22.0846335516218,2.58536692026875,7.45365185399615));
#45834=CARTESIAN_POINT('Ctrl Pts',(21.9263792420531,-0.725690223623306,
6.44452750096693));
#45835=CARTESIAN_POINT('Ctrl Pts',(21.7681249324843,-3.37644964973648,8.67048927925364));
#45836=CARTESIAN_POINT('Ctrl Pts',(21.6098706229155,-2.95501390620346,12.1061585427555));
#45837=CARTESIAN_POINT('Ctrl Pts',(21.4516163133467,0.155157162744094,13.6254568329877));
#45838=CARTESIAN_POINT('Ctrl Pts',(21.2933620037779,3.1241524005353,11.845990999834));
#45839=CARTESIAN_POINT('Ctrl Pts',(21.1351076942091,3.2505150185073,8.38687783860446));
#45840=CARTESIAN_POINT('Ctrl Pts',(20.9768533846404,0.419269031639233,6.39552715751162));
#45841=CARTESIAN_POINT('Ctrl Pts',(20.8185990750715,-2.79346533128499,7.6838474929171));
#45842=CARTESIAN_POINT('Ctrl Pts',(20.6603447655028,-3.46445567698268,11.0796100478242));
#45843=CARTESIAN_POINT('Ctrl Pts',(20.502090455934,-0.983175116979502,13.4930470484227));
#45844=CARTESIAN_POINT('Ctrl Pts',(20.3438361463652,2.39268589243202,12.7281981623963));
#45845=CARTESIAN_POINT('Ctrl Pts',(20.1855818367964,3.59146777933862,9.48099115314302));
#45846=CARTESIAN_POINT('Ctrl Pts',(20.0273275272277,1.52241181662405,6.70602470353113));
#45847=CARTESIAN_POINT('Ctrl Pts',(19.8690732176588,-1.93187026052108,6.9282108975943));
#45848=CARTESIAN_POINT('Ctrl Pts',(19.7108189080901,-3.62836439530803,9.94538491046653));
#45849=CARTESIAN_POINT('Ctrl Pts',(19.5525645985213,-2.02344884700714,13.0122526050597));
#45850=CARTESIAN_POINT('Ctrl Pts',(19.3943102889525,1.42258101312554,13.3383040985265));
#45851=CARTESIAN_POINT('Ctrl Pts',(19.2360559793837,3.57421973167857,10.6268686487801));
#45852=CARTESIAN_POINT('Ctrl Pts',(19.0778016698149,2.47371441340158,7.34505216735374));
#45853=CARTESIAN_POINT('Ctrl Pts',(18.9195473602461,-0.877597005871997,
6.47894412307493));
#45854=CARTESIAN_POINT('Ctrl Pts',(18.7612930506773,-3.43039236187988,8.81660689680056));
#45855=CARTESIAN_POINT('Ctrl Pts',(18.6030387411086,-2.86191065570903,12.231026309097));
#45856=CARTESIAN_POINT('Ctrl Pts',(18.4447844315398,0.31059273116958,13.6154589125709));
#45857=CARTESIAN_POINT('Ctrl Pts',(18.286530121971,3.2004911372734,11.7102243926977));
#45858=CARTESIAN_POINT('Ctrl Pts',(18.1282758124023,3.17829712925949,8.24887511830688));
#45859=CARTESIAN_POINT('Ctrl Pts',(17.9700215028334,0.264204795973602,6.38085551284168));
#45860=CARTESIAN_POINT('Ctrl Pts',(17.8117671932647,-2.89028463548505,7.80585649534429));
#45861=CARTESIAN_POINT('Ctrl Pts',(17.6535128836959,-3.41493520764679,11.2272850201637));
#45862=CARTESIAN_POINT('Ctrl Pts',(17.4952585741271,-0.832373015781326,
13.5320201239153));
#45863=CARTESIAN_POINT('Ctrl Pts',(17.3370042645583,2.50755641786257,12.6230081594193));
#45864=CARTESIAN_POINT('Ctrl Pts',(17.1787499549895,3.56588727515458,9.32734932243063));
#45865=CARTESIAN_POINT('Ctrl Pts',(17.0204956454207,1.37965570806092,6.64372809201059));
#45866=CARTESIAN_POINT('Ctrl Pts',(16.862241335852,-2.06190972787176,7.0139425211072));
#45867=CARTESIAN_POINT('Ctrl Pts',(16.7039870262831,-3.62736571072646,10.1011384881722));
#45868=CARTESIAN_POINT('Ctrl Pts',(16.5457327167144,-1.89232070283748,13.0963096341866));
#45869=CARTESIAN_POINT('Ctrl Pts',(16.3874784071456,1.56452653085165,13.2741819936291));
#45870=CARTESIAN_POINT('Ctrl Pts',(16.2292240975768,3.59782792524174,10.4729114224616));
#45871=CARTESIAN_POINT('Ctrl Pts',(16.070969788008,2.35750444175658,7.24134384160661));
#45872=CARTESIAN_POINT('Ctrl Pts',(15.9127154784392,-1.02788694119381,6.51984778648015));
#45873=CARTESIAN_POINT('Ctrl Pts',(15.7544611688705,-3.4780150674644,8.96490474658875));
#45874=CARTESIAN_POINT('Ctrl Pts',(15.5962068593017,-2.76353474467712,12.3517837290249));
#45875=CARTESIAN_POINT('Ctrl Pts',(15.4379525497329,0.465456076952267,13.598800026894));
#45876=CARTESIAN_POINT('Ctrl Pts',(15.2796982401641,3.27093342747344,11.5713069420647));
#45877=CARTESIAN_POINT('Ctrl Pts',(15.1214439305953,3.10022368274011,8.11409859480372));
#45878=CARTESIAN_POINT('Ctrl Pts',(14.9631896210265,0.108653800813268,6.37285162355982));
#45879=CARTESIAN_POINT('Ctrl Pts',(14.8049353114577,-2.98177900419071,7.93190789293335));
#45880=CARTESIAN_POINT('Ctrl Pts',(14.6466810018889,-3.35912320927538,11.3726988956255));
#45881=CARTESIAN_POINT('Ctrl Pts',(14.4884266923202,-0.680037386513999,
13.5644859581834));
#45882=CARTESIAN_POINT('Ctrl Pts',(14.3301723827514,2.61780712972438,12.5129856395747));
#45883=CARTESIAN_POINT('Ctrl Pts',(14.1719180731826,3.53373713437049,9.17494675425479));
#45884=CARTESIAN_POINT('Ctrl Pts',(14.0136637636138,1.23435778144942,6.58761493079715));
#45885=CARTESIAN_POINT('Ctrl Pts',(13.855409454045,-2.18815042185467,7.10517552786303));
#45886=CARTESIAN_POINT('Ctrl Pts',(13.6971551444763,-3.61968412433208,10.2567057326988));
#45887=CARTESIAN_POINT('Ctrl Pts',(13.5389008349074,-1.75770622879056,13.1746621562634));
#45888=CARTESIAN_POINT('Ctrl Pts',(13.3806465253387,1.70358963251637,13.2040276773368));
#45889=CARTESIAN_POINT('Ctrl Pts',(13.2223922157699,3.6148076361298,10.3180829245743));
#45890=CARTESIAN_POINT('Ctrl Pts',(13.0641379062011,2.23695110582196,7.14271794474384));
#45891=CARTESIAN_POINT('Ctrl Pts',(12.9058835966323,-1.17628314204709,6.5671631319018));
#45892=CARTESIAN_POINT('Ctrl Pts',(12.7476292870635,-3.51923002839292,9.11510961115741));
#45893=CARTESIAN_POINT('Ctrl Pts',(12.5893749774948,-2.66006741669669,12.4682083242114));
#45894=CARTESIAN_POINT('Ctrl Pts',(12.431120667926,0.619461886626625,13.5755108676666));
#45895=CARTESIAN_POINT('Ctrl Pts',(12.2728663583572,3.33534949119645,11.4294945832771));
#45896=CARTESIAN_POINT('Ctrl Pts',(12.1146120487884,3.01643851828712,7.98279657484158));
#45897=CARTESIAN_POINT('Ctrl Pts',(11.9563577392196,-0.047097373778369,
6.37153023510597));
#45898=CARTESIAN_POINT('Ctrl Pts',(11.7981034296508,-3.06777987142775,8.06176945515013));
#45899=CARTESIAN_POINT('Ctrl Pts',(11.639849120082,-3.2971225088352,11.5155837678287));
#45900=CARTESIAN_POINT('Ctrl Pts',(11.4815948105133,-0.526448883152259,
13.5903847416995));
#45901=CARTESIAN_POINT('Ctrl Pts',(11.3233405009445,2.72323490185543,12.3983332956597));
#45902=CARTESIAN_POINT('Ctrl Pts',(11.1650861913757,3.49507659867442,9.02406424380673));
#45903=CARTESIAN_POINT('Ctrl Pts',(11.0068318818069,1.08678570881093,6.53778857091659));
#45904=CARTESIAN_POINT('Ctrl Pts',(10.8485775722381,-2.31035972625494,7.20174189080126));
#45905=CARTESIAN_POINT('Ctrl Pts',(10.6903232626693,-3.60533385732009,10.411799924513));
#45906=CARTESIAN_POINT('Ctrl Pts',(10.5320689531006,-1.61985329993334,13.2471660282134));
#45907=CARTESIAN_POINT('Ctrl Pts',(10.3738146435318,1.83951385849227,13.127969994097));
#45908=CARTESIAN_POINT('Ctrl Pts',(10.215560333963,3.62512807421833,10.1626691840488));
#45909=CARTESIAN_POINT('Ctrl Pts',(10.0573060243942,2.11227555931511,7.04935467956235));
#45910=CARTESIAN_POINT('Ctrl Pts',(9.89905171482542,-1.32251038305822,6.62080587867383));
#45911=CARTESIAN_POINT('Ctrl Pts',(9.74079740525663,-3.55396482958843,9.2669391921202));
#45912=CARTESIAN_POINT('Ctrl Pts',(9.58254309568785,-2.55169252158856,12.5800963203793));
#45913=CARTESIAN_POINT('Ctrl Pts',(9.42428878611906,0.772313381832412,13.5456136953941));
#45914=CARTESIAN_POINT('Ctrl Pts',(9.26603447655028,3.39364577165048,11.2850883447562));
#45915=CARTESIAN_POINT('Ctrl Pts',(9.1077801669815,2.92704762252235,7.85513439723516));
#45916=CARTESIAN_POINT('Ctrl Pts',(8.94952585741271,-0.20266861905204,6.37704123220448));
#45917=CARTESIAN_POINT('Ctrl Pts',(8.79127154784393,-3.14830820588747,8.19491794102147));
#45918=CARTESIAN_POINT('Ctrl Pts',(8.63301723827514,-3.22870170972224,11.6562236610067));
#45919=CARTESIAN_POINT('Ctrl Pts',(8.47476292870636,-0.372557211312175,
13.6086112664375));
#45920=CARTESIAN_POINT('Ctrl Pts',(8.31650861913757,2.82494041479191,12.281332723926));
#45921=CARTESIAN_POINT('Ctrl Pts',(8.15825430956879,3.44737991946778,8.87067395584943));
#45922=CARTESIAN_POINT('Ctrl Pts',(8.05275143652293,1.7779394739971,7.29387947745118));
#45923=CARTESIAN_POINT('Ctrl Pts',(8.,0.793799282532855,7.0307770462543));
#45924=CARTESIAN_POINT('Ctrl Pts',(25.8782388507408,2.51331533716111,9.85490600980487));
#45925=CARTESIAN_POINT('Ctrl Pts',(25.8769239147893,2.52685451631763,9.54765567369101));
#45926=CARTESIAN_POINT('Ctrl Pts',(25.8804442384711,2.49183285130677,9.23944408489687));
#45927=CARTESIAN_POINT('Ctrl Pts',(25.8965480296803,2.31890412387178,8.60639456830937));
#45928=CARTESIAN_POINT('Ctrl Pts',(25.9101919837067,2.16864405658939,8.28772728731036));
#45929=CARTESIAN_POINT('Ctrl Pts',(25.9371024584265,1.81388157912996,7.7895766632932));
#45930=CARTESIAN_POINT('Ctrl Pts',(25.9495040585495,1.63266221909673,7.59663063038989));
#45931=CARTESIAN_POINT('Ctrl Pts',(25.9737270380795,1.19204230912881,7.24399771550759));
#45932=CARTESIAN_POINT('Ctrl Pts',(25.9849858624053,0.928010439591528,7.09546117333466));
#45933=CARTESIAN_POINT('Ctrl Pts',(25.9920223077014,0.644031331499198,6.99473364008323));
#45934=CARTESIAN_POINT('Ctrl Pts',(24.387416697508,-2.51385573226095,9.99896352468483));
#45935=CARTESIAN_POINT('Ctrl Pts',(24.4095944865459,-2.51517282451638,9.64697137526858));
#45936=CARTESIAN_POINT('Ctrl Pts',(24.4317722755838,-2.44620577848239,9.29547212983497));
#45937=CARTESIAN_POINT('Ctrl Pts',(24.4539500646217,-2.30443020970175,8.97631530577795));
#45938=CARTESIAN_POINT('Ctrl Pts',(24.5067015011447,-1.96720701291458,8.21717827384355));
#45939=CARTESIAN_POINT('Ctrl Pts',(24.5594529376676,-1.2180624633474,7.64102166045144));
#45940=CARTESIAN_POINT('Ctrl Pts',(24.6122043741905,-0.397791013133248,
7.50998874563856));
#45941=CARTESIAN_POINT('Ctrl Pts',(24.6649558107135,0.422480437080906,7.37895583082568));
#45942=CARTESIAN_POINT('Ctrl Pts',(24.7177072472364,1.31387878794203,7.69304661459202));
#45943=CARTESIAN_POINT('Ctrl Pts',(24.7704586837593,1.87081935093645,8.30932110024717));
#45944=CARTESIAN_POINT('Ctrl Pts',(24.8232101202822,2.42775991393086,8.92559558590231));
#45945=CARTESIAN_POINT('Ctrl Pts',(24.8759615568051,2.65024268905857,9.84405377344627));
#45946=CARTESIAN_POINT('Ctrl Pts',(24.9287129933281,2.43714240994448,10.6469368095826));
#45947=CARTESIAN_POINT('Ctrl Pts',(24.981464429851,2.2240421308304,11.4498198457189));
#45948=CARTESIAN_POINT('Ctrl Pts',(25.034215866374,1.57535879747453,12.1371277304477));
#45949=CARTESIAN_POINT('Ctrl Pts',(25.0869673028969,0.786030030008762,12.3960024953926));
#45950=CARTESIAN_POINT('Ctrl Pts',(25.1397187394198,-0.00329873745700912,
12.6548772603375));
#45951=CARTESIAN_POINT('Ctrl Pts',(25.1924701759427,-0.933272939032685,
12.4853189054987));
#45952=CARTESIAN_POINT('Ctrl Pts',(25.2452216124657,-1.58046369528845,11.964796607642));
#45953=CARTESIAN_POINT('Ctrl Pts',(25.2926199741465,-2.16197926270129,11.4970955218905));
#45954=CARTESIAN_POINT('Ctrl Pts',(25.3400183358272,-2.51519159740436,10.7460461564513));
#45955=CARTESIAN_POINT('Ctrl Pts',(25.387416697508,-2.52031926711485,9.99879747833012));
#45956=CARTESIAN_POINT('Ctrl Pts',(8.,0.793799282532855,7.0307770462543));
#45957=CARTESIAN_POINT('Ctrl Pts',(8.,0.888651840235432,7.06547453556552));
#45958=CARTESIAN_POINT('Ctrl Pts',(8.00000000000001,0.981460615688964,7.10515936495498));
#45959=CARTESIAN_POINT('Ctrl Pts',(8.00000000000001,1.071984630131,7.14951198682703));
#45960=CARTESIAN_POINT('Ctrl Pts',(8.00000000000001,1.16377090416436,7.19448305809844));
#45961=CARTESIAN_POINT('Ctrl Pts',(8.,1.25320892391096,7.24425370524276));
#45962=CARTESIAN_POINT('Ctrl Pts',(8.,1.3400134543598,7.29853149073832));
#45963=CARTESIAN_POINT('Ctrl Pts',(8.,1.36448894626115,7.31383570922151));
#45964=CARTESIAN_POINT('Ctrl Pts',(8.,1.38875483117205,7.32949846326485));
#45965=CARTESIAN_POINT('Ctrl Pts',(8.,1.41280412179919,7.34551365083284));
#45966=CARTESIAN_POINT('Ctrl Pts',(8.,1.43214636521133,7.3583942659426));
#45967=CARTESIAN_POINT('Ctrl Pts',(8.00000000000001,1.45135061788146,7.37150448852873));
#45968=CARTESIAN_POINT('Ctrl Pts',(8.00000000000001,1.47039392887492,7.38482736395197));
#45969=CARTESIAN_POINT('Ctrl Pts',(8.00000000000001,1.55310526312923,7.44269297370535));
#45970=CARTESIAN_POINT('Ctrl Pts',(8.00000000000001,1.63286195332271,7.50461801758942));
#45971=CARTESIAN_POINT('Ctrl Pts',(8.00000000000001,1.70939770627191,7.570306093392));
#45972=CARTESIAN_POINT('Ctrl Pts',(8.00000000000001,1.76856435887146,7.62108685154987));
#45973=CARTESIAN_POINT('Ctrl Pts',(8.00000000000001,1.82580548371507,7.67411738544499));
#45974=CARTESIAN_POINT('Ctrl Pts',(8.00000000000001,1.8809803115492,7.72927264183758));
#45975=CARTESIAN_POINT('Ctrl Pts',(8.00000000000001,1.91054892908599,7.75883077088729));
#45976=CARTESIAN_POINT('Ctrl Pts',(8.00000000000001,1.93952383038483,7.78899926613622));
#45977=CARTESIAN_POINT('Ctrl Pts',(8.00000000000001,1.96788125663504,7.81975974016046));
#45978=CARTESIAN_POINT('Ctrl Pts',(8.00000000000001,1.97854463399386,7.8313267469601));
#45979=CARTESIAN_POINT('Ctrl Pts',(8.00000000000001,1.98911861632425,7.84297530088787));
#45980=CARTESIAN_POINT('Ctrl Pts',(8.00000000000001,1.99959529223268,7.85469662340685));
#45981=CARTESIAN_POINT('Ctrl Pts',(8.00000000000001,2.06523110597061,7.92813008153257));
#45982=CARTESIAN_POINT('Ctrl Pts',(8.,2.12713067340333,8.00450310115816));
#45983=CARTESIAN_POINT('Ctrl Pts',(8.,2.18504938463886,8.08353870982025));
#45984=CARTESIAN_POINT('Ctrl Pts',(8.,2.24239481491336,8.16179202190283));
#45985=CARTESIAN_POINT('Ctrl Pts',(8.00000000000001,2.29583822969202,8.24265625774018));
#45986=CARTESIAN_POINT('Ctrl Pts',(8.00000000000001,2.34509645146655,8.32588467382346));
#45987=CARTESIAN_POINT('Ctrl Pts',(8.00000000000001,2.39296142701126,8.40675901229807));
#45988=CARTESIAN_POINT('Ctrl Pts',(8.,2.43687482302416,8.48986637651382));
#45989=CARTESIAN_POINT('Ctrl Pts',(8.,2.47652901207894,8.57499049794785));
#45990=CARTESIAN_POINT('Ctrl Pts',(8.,2.49722179256097,8.61941089338518));
#45991=CARTESIAN_POINT('Ctrl Pts',(8.,2.51675394122296,8.66438057335268));
#45992=CARTESIAN_POINT('Ctrl Pts',(8.,2.53507605865623,8.70986902566855));
#45993=CARTESIAN_POINT('Ctrl Pts',(8.,2.54220474646394,8.72756746999938));
#45994=CARTESIAN_POINT('Ctrl Pts',(8.00000000000001,2.54915021624124,8.74534444465406));
#45995=CARTESIAN_POINT('Ctrl Pts',(8.00000000000001,2.55590938804843,8.76319814293423));
#45996=CARTESIAN_POINT('Ctrl Pts',(8.00000000000001,2.56088080950049,8.77632967164225));
#45997=CARTESIAN_POINT('Ctrl Pts',(8.00000000000001,2.565750374188,8.78950002479304));
#45998=CARTESIAN_POINT('Ctrl Pts',(8.00000000000001,2.57051357424907,8.80269860187458));
#45999=CARTESIAN_POINT('Ctrl Pts',(8.00000000000001,2.60204053185424,8.89005814477923));
#46000=CARTESIAN_POINT('Ctrl Pts',(8.00000000000001,2.62895893279742,8.97877679643224));
#46001=CARTESIAN_POINT('Ctrl Pts',(8.00000000000001,2.65101703259939,9.06863225769505));
#46002=CARTESIAN_POINT('Ctrl Pts',(8.00000000000001,2.65603223898398,9.08906210827427));
#46003=CARTESIAN_POINT('Ctrl Pts',(8.,2.66079598776046,9.10955076534661));
#46004=CARTESIAN_POINT('Ctrl Pts',(8.,2.66530494352163,9.13009567307715));
#46005=CARTESIAN_POINT('Ctrl Pts',(8.,2.68549215663049,9.22207804164026));
#46006=CARTESIAN_POINT('Ctrl Pts',(8.,2.70057625721049,9.31518827802502));
#46007=CARTESIAN_POINT('Ctrl Pts',(8.,2.71066780876488,9.40903345925902));
#46008=CARTESIAN_POINT('Ctrl Pts',(8.,2.7212185892897,9.50714918558466));
#46009=CARTESIAN_POINT('Ctrl Pts',(8.,2.72631209524207,9.60606952165998));
#46010=CARTESIAN_POINT('Ctrl Pts',(8.,2.72601695513705,9.70533038478544));
#46011=CARTESIAN_POINT('Ctrl Pts',(8.,2.72591332999743,9.74018136106902));
#46012=CARTESIAN_POINT('Ctrl Pts',(8.00000000000001,2.72514492076099,9.77507409305378));
#46013=CARTESIAN_POINT('Ctrl Pts',(8.00000000000001,2.72371312681726,9.80998762211471));
#46014=CARTESIAN_POINT('Ctrl Pts',(8.00000000000001,2.72312104730935,9.82442516405044));
#46015=CARTESIAN_POINT('Ctrl Pts',(8.,2.72241541659262,9.83886678055821));
#46016=CARTESIAN_POINT('Ctrl Pts',(8.,2.72159739125326,9.85329547547575));
#46017=CARTESIAN_POINT('Ctrl Pts',(8.,2.71633099801499,9.9461864627038));
#46018=CARTESIAN_POINT('Ctrl Pts',(8.,2.70640503210548,10.0386981093905));
#46019=CARTESIAN_POINT('Ctrl Pts',(8.,2.69194454036193,10.1304577877966));
#46020=CARTESIAN_POINT('Ctrl Pts',(8.,2.67751755146885,10.2220048724098));
#46021=CARTESIAN_POINT('Ctrl Pts',(8.,2.65857661117198,10.3128044168814));
#46022=CARTESIAN_POINT('Ctrl Pts',(8.,2.63519721280128,10.4024694307445));
#46023=CARTESIAN_POINT('Ctrl Pts',(8.,2.61221588141411,10.4906077722342));
#46024=CARTESIAN_POINT('Ctrl Pts',(8.,2.58494547647907,10.5776506751394));
#46025=CARTESIAN_POINT('Ctrl Pts',(8.,2.55341730266435,10.663201462517));
#46026=CARTESIAN_POINT('Ctrl Pts',(8.,2.53742523481517,10.7065954758949));
#46027=CARTESIAN_POINT('Ctrl Pts',(8.,2.52033710900699,10.7496050527093));
#46028=CARTESIAN_POINT('Ctrl Pts',(8.,2.50215350356533,10.792174520464));
#46029=CARTESIAN_POINT('Ctrl Pts',(8.,2.49664128219483,10.8050791300939));
#46030=CARTESIAN_POINT('Ctrl Pts',(8.00000000000001,2.49102837597118,10.8179432750348));
#46031=CARTESIAN_POINT('Ctrl Pts',(8.00000000000001,2.48531476150017,10.830765348423));
#46032=CARTESIAN_POINT('Ctrl Pts',(8.00000000000001,2.47974569525222,10.8432630373198));
#46033=CARTESIAN_POINT('Ctrl Pts',(8.,2.47408470333919,10.8557123142945));
#46034=CARTESIAN_POINT('Ctrl Pts',(8.,2.46833291255443,10.8681102233784));
#46035=CARTESIAN_POINT('Ctrl Pts',(8.,2.43083362022605,10.948939452812));
#46036=CARTESIAN_POINT('Ctrl Pts',(8.,2.38946742072689,11.0276121176187));
#46037=CARTESIAN_POINT('Ctrl Pts',(8.,2.34430545470983,11.1037797259104));
#46038=CARTESIAN_POINT('Ctrl Pts',(8.,2.29990596796576,11.1786613799419));
#46039=CARTESIAN_POINT('Ctrl Pts',(8.,2.25183734528232,11.2511225203992));
#46040=CARTESIAN_POINT('Ctrl Pts',(8.,2.20013104971758,11.3207978239273));
#46041=CARTESIAN_POINT('Ctrl Pts',(8.,2.15002363316517,11.3883186048915));
#46042=CARTESIAN_POINT('Ctrl Pts',(8.,2.09649959036919,11.4532236127033));
#46043=CARTESIAN_POINT('Ctrl Pts',(8.,2.03955998698964,11.5151401317574));
#46044=CARTESIAN_POINT('Ctrl Pts',(8.,2.01641826334308,11.5403046023203));
#46045=CARTESIAN_POINT('Ctrl Pts',(8.,1.99271206342713,11.5649749200134));
#46046=CARTESIAN_POINT('Ctrl Pts',(8.,1.9684403447054,11.5891238290966));
#46047=CARTESIAN_POINT('Ctrl Pts',(8.,1.95158317542738,11.6058957047499));
#46048=CARTESIAN_POINT('Ctrl Pts',(8.,1.93445320326802,11.622416041126));
#46049=CARTESIAN_POINT('Ctrl Pts',(8.,1.91705735205381,11.6386813803728));
#46050=CARTESIAN_POINT('Ctrl Pts',(25.7084234471775,-3.07694191359583,9.99853189658296));
#46051=CARTESIAN_POINT('Ctrl Pts',(25.6610250854967,-3.07068177740707,10.9108134505871));
#46052=CARTESIAN_POINT('Ctrl Pts',(25.560875287293,-2.15953918737736,12.8482119976726));
#46053=CARTESIAN_POINT('Ctrl Pts',(25.4079740525663,1.13133546731627,13.4482235802362));
#46054=CARTESIAN_POINT('Ctrl Pts',(25.2497197429975,3.5071784366143,10.9309157942814));
#46055=CARTESIAN_POINT('Ctrl Pts',(25.0914654334287,2.69232146419524,7.56700567779718));
#46056=CARTESIAN_POINT('Ctrl Pts',(24.93321112386,-0.572480320954722,6.41662868803847));
#46057=CARTESIAN_POINT('Ctrl Pts',(24.8055304617762,-2.7861876229203,8.119160065833));
#46058=CARTESIAN_POINT('Ctrl Pts',(24.7306012362154,-3.07065885845128,9.56900358366952));
#46059=CARTESIAN_POINT('Ctrl Pts',(24.7084234471775,-3.06905088107409,9.99873461494295));
#46060=CARTESIAN_POINT('Origin',(28.2084234471774,0.,10.));
#46061=CARTESIAN_POINT('Ctrl Pts',(25.7915765528226,-3.07002654794609,10.0000640341964));
#46062=CARTESIAN_POINT('Ctrl Pts',(25.7505300621955,-3.06421617930135,10.7929818643657));
#46063=CARTESIAN_POINT('Ctrl Pts',(25.6568828586135,-2.35442447610646,12.6045285619815));
#46064=CARTESIAN_POINT('Ctrl Pts',(25.5106349420764,0.701596196644071,13.5590880549712));
#46065=CARTESIAN_POINT('Ctrl Pts',(25.3528328032114,3.3594675732725,11.3600672948067));
#46066=CARTESIAN_POINT('Ctrl Pts',(25.1950306643464,2.97881274377391,7.93379586486837));
#46067=CARTESIAN_POINT('Ctrl Pts',(25.0372285254814,-0.0991962456131474,
6.3757557658597));
#46068=CARTESIAN_POINT('Ctrl Pts',(24.9027438216401,-2.64536456776374,7.84448501581014));
#46069=CARTESIAN_POINT('Ctrl Pts',(24.8208598307538,-3.06731791981827,9.43344524461191));
#46070=CARTESIAN_POINT('Ctrl Pts',(24.7915765528225,-3.06884999403827,10.0009308069803));
#46071=CARTESIAN_POINT('Ctrl Pts',(25.8262392198064,-3.0008944935354,9.33589572455155));
#46072=CARTESIAN_POINT('Ctrl Pts',(25.7736385068514,-3.22038097435984,10.3276914350471));
#46073=CARTESIAN_POINT('Ctrl Pts',(25.6684370809415,-2.59586341847174,12.5291142048513));
#46074=CARTESIAN_POINT('Ctrl Pts',(25.5106349420764,0.701596196644071,13.5590880549712));
#46075=CARTESIAN_POINT('Ctrl Pts',(25.3528328032114,3.3594675732725,11.3600672948067));
#46076=CARTESIAN_POINT('Ctrl Pts',(25.1950306643464,2.97881274377391,7.93379586486837));
#46077=CARTESIAN_POINT('Ctrl Pts',(25.0372285254814,-0.0991962456131474,
6.3757557658597));
#46078=CARTESIAN_POINT('Ctrl Pts',(24.8794263866164,-3.08682826374848,8.09913850334405));
#46079=CARTESIAN_POINT('Ctrl Pts',(24.7216242477514,-3.28078721105507,11.5425223969915));
#46080=CARTESIAN_POINT('Ctrl Pts',(24.5638221088864,-0.505048782495192,
13.5899960272459));
#46081=CARTESIAN_POINT('Ctrl Pts',(24.4060199700213,2.72774157840345,12.387916003312));
#46082=CARTESIAN_POINT('Ctrl Pts',(24.2482178311564,3.49161491002287,9.0245357108578));
#46083=CARTESIAN_POINT('Ctrl Pts',(24.0904156922914,1.09510149634942,6.54403898763965));
#46084=CARTESIAN_POINT('Ctrl Pts',(23.9326135534264,-2.29260925396287,7.19165511461472));
#46085=CARTESIAN_POINT('Ctrl Pts',(23.7748114145613,-3.60521723307181,10.3811773897178));
#46086=CARTESIAN_POINT('Ctrl Pts',(23.6170092756964,-1.65463280838614,13.2256900191163));
#46087=CARTESIAN_POINT('Ctrl Pts',(23.4592071368313,1.79360733424122,13.1505319563297));
#46088=CARTESIAN_POINT('Ctrl Pts',(23.3014049979663,3.61840100535183,10.2237352102483));
#46089=CARTESIAN_POINT('Ctrl Pts',(23.1436028591013,2.16807193309428,7.09442832744505));
#46090=CARTESIAN_POINT('Ctrl Pts',(22.9858007202363,-1.24464326464773,6.59504112130271));
#46091=CARTESIAN_POINT('Ctrl Pts',(22.8279985813713,-3.53079496446001,9.17758320677621));
#46092=CARTESIAN_POINT('Ctrl Pts',(22.6701964425063,-2.62111912833757,12.5045192826475));
#46093=CARTESIAN_POINT('Ctrl Pts',(22.5123943036413,0.661009511544134,13.5645404549472));
#46094=CARTESIAN_POINT('Ctrl Pts',(22.3545921647763,3.34483881058325,11.3981901341401));
#46095=CARTESIAN_POINT('Ctrl Pts',(22.1967900259113,3.0011550686756,7.96629634724844));
#46096=CARTESIAN_POINT('Ctrl Pts',(22.0389878870462,-0.0589633304184637,
6.37516819565949));
#46097=CARTESIAN_POINT('Ctrl Pts',(21.8811857481813,-3.06571226878003,8.06498305391951));
#46098=CARTESIAN_POINT('Ctrl Pts',(21.7233836093162,-3.29759390354424,11.5062392702711));
#46099=CARTESIAN_POINT('Ctrl Pts',(21.5655814704513,-0.544725276252224,
13.5841535492561));
#46100=CARTESIAN_POINT('Ctrl Pts',(21.4077793315862,2.70119039079158,12.4179439128307));
#46101=CARTESIAN_POINT('Ctrl Pts',(21.2499771927212,3.50217834240436,9.06318136752485));
#46102=CARTESIAN_POINT('Ctrl Pts',(21.0921750538562,1.13324057456603,6.55636121344182));
#46103=CARTESIAN_POINT('Ctrl Pts',(20.9343729149912,-2.26142692279634,7.16648088674201));
#46104=CARTESIAN_POINT('Ctrl Pts',(20.7765707761262,-3.60920969167029,10.3413029355054));
#46105=CARTESIAN_POINT('Ctrl Pts',(20.6187686372612,-1.69018948530375,13.2072015521334));
#46106=CARTESIAN_POINT('Ctrl Pts',(20.4609664983962,1.75867146489572,13.1701667102578));
#46107=CARTESIAN_POINT('Ctrl Pts',(20.3031643595312,3.61570659591804,10.2637197460999));
#46108=CARTESIAN_POINT('Ctrl Pts',(20.1453622206662,2.20005821053506,7.11857220071228));
#46109=CARTESIAN_POINT('Ctrl Pts',(19.9875600818011,-1.20692825766852,6.58149060655154));
#46110=CARTESIAN_POINT('Ctrl Pts',(19.8297579429362,-3.52148808405926,9.13860347918041));
#46111=CARTESIAN_POINT('Ctrl Pts',(19.6719558040711,-2.64864436976049,12.4753919477101));
#46112=CARTESIAN_POINT('Ctrl Pts',(19.5141536652062,0.621566094242422,13.5716295836412));
#46113=CARTESIAN_POINT('Ctrl Pts',(19.3563515263411,3.32917861036942,11.4350791171607));
#46114=CARTESIAN_POINT('Ctrl Pts',(19.1985493874761,3.02345260681924,7.99959588418488));
#46115=CARTESIAN_POINT('Ctrl Pts',(19.0407472486111,-0.0188902229263912,
6.37473787820383));
#46116=CARTESIAN_POINT('Ctrl Pts',(18.8829451097461,-3.04413495039173,8.03121237913899));
#46117=CARTESIAN_POINT('Ctrl Pts',(18.7251429708811,-3.31404264771403,11.4696950776895));
#46118=CARTESIAN_POINT('Ctrl Pts',(18.5673408320161,-0.584311835073177,
13.5779130749147));
#46119=CARTESIAN_POINT('Ctrl Pts',(18.4095386931511,2.6742969880911,12.4476555950008));
#46120=CARTESIAN_POINT('Ctrl Pts',(18.2517365542861,3.51232011417934,9.10195227978501));
#46121=CARTESIAN_POINT('Ctrl Pts',(18.0939344154211,1.17123790163294,6.56909865049566));
#46122=CARTESIAN_POINT('Ctrl Pts',(17.9361322765561,-2.22996655058651,7.14165581577071));
#46123=CARTESIAN_POINT('Ctrl Pts',(17.7783301376911,-3.6127619923839,10.3013852661271));
#46124=CARTESIAN_POINT('Ctrl Pts',(17.6205279988261,-1.72553916596101,13.1883219534713));
#46125=CARTESIAN_POINT('Ctrl Pts',(17.462725859961,1.72352045101636,13.1894136682438));
#46126=CARTESIAN_POINT('Ctrl Pts',(17.3049237210961,3.61257047634171,10.3036722669531));
#46127=CARTESIAN_POINT('Ctrl Pts',(17.147121582231,2.23177558030935,7.14306807022165));
#46128=CARTESIAN_POINT('Ctrl Pts',(16.989319443366,-1.1690657327204,6.56835788508897));
#46129=CARTESIAN_POINT('Ctrl Pts',(16.831517304501,-3.5117509007273,9.09972898330938));
#46130=CARTESIAN_POINT('Ctrl Pts',(16.673715165636,-2.67584594211482,12.4459621391836));
#46131=CARTESIAN_POINT('Ctrl Pts',(16.515913026771,0.582046717903019,13.5782822569538));
#46132=CARTESIAN_POINT('Ctrl Pts',(16.358110887906,3.3131115922785,11.4717927399475));
#46133=CARTESIAN_POINT('Ctrl Pts',(16.200308749041,3.04538068264102,8.03313986515331));
#46134=CARTESIAN_POINT('Ctrl Pts',(16.042506610176,0.0211851935724078,6.37475056308874));
#46135=CARTESIAN_POINT('Ctrl Pts',(15.884704471311,-3.02218564392591,7.99768228647392));
#46136=CARTESIAN_POINT('Ctrl Pts',(15.7269023324459,-3.33008642100386,11.4329712910236));
#46137=CARTESIAN_POINT('Ctrl Pts',(15.569100193581,-0.623826992014808,13.5712353851694));
#46138=CARTESIAN_POINT('Ctrl Pts',(15.4112980547159,2.6470767906288,12.4770681776581));
#46139=CARTESIAN_POINT('Ctrl Pts',(15.2534959158509,3.52203268603658,9.14083293199628));
#46140=CARTESIAN_POINT('Ctrl Pts',(15.0956937769859,1.20909210531671,6.58225533822185));
#46141=CARTESIAN_POINT('Ctrl Pts',(14.9378916381209,-2.19823368004202,7.11718002986987));
#46142=CARTESIAN_POINT('Ctrl Pts',(14.7800894992559,-3.61587281936424,10.2614307679579));
#46143=CARTESIAN_POINT('Ctrl Pts',(14.6222873603909,-1.76067798849733,13.1690527469692));
#46144=CARTESIAN_POINT('Ctrl Pts',(14.4644852215259,1.68815882569895,13.2082708849888));
#46145=CARTESIAN_POINT('Ctrl Pts',(14.3066830826609,3.60899290643803,10.3435876795407));
#46146=CARTESIAN_POINT('Ctrl Pts',(14.1488809437959,2.26322023068206,7.16791305223806));
#46147=CARTESIAN_POINT('Ctrl Pts',(13.9910788049309,-1.13106034981207,6.55564450479696));
#46148=CARTESIAN_POINT('Ctrl Pts',(13.8332766660659,-3.50158458705909,9.06096449911507));
#46149=CARTESIAN_POINT('Ctrl Pts',(13.6754745272009,-2.70272053038027,12.4162334380006));
#46150=CARTESIAN_POINT('Ctrl Pts',(13.5176723883359,0.542456216386849,13.5844976699054));
#46151=CARTESIAN_POINT('Ctrl Pts',(13.3598702494708,3.2966397172568,11.5083265120178));
#46152=CARTESIAN_POINT('Ctrl Pts',(13.2020681106059,3.06693661782036,8.06692419328139));
#46153=CARTESIAN_POINT('Ctrl Pts',(13.0442659717408,0.0612580212745303,
6.37520624764731));
#46154=CARTESIAN_POINT('Ctrl Pts',(12.8864638328758,-2.99986703121441,7.96439687383041));
#46155=CARTESIAN_POINT('Ctrl Pts',(12.7286616940108,-3.34572326306573,11.396072397554));
#46156=CARTESIAN_POINT('Ctrl Pts',(12.5708595551458,-0.663265918297566,
13.5641212961923));
#46157=CARTESIAN_POINT('Ctrl Pts',(12.4130574162808,2.61953312462283,12.5061780665257));
#46158=CARTESIAN_POINT('Ctrl Pts',(12.2552552774158,3.53131487113802,9.17981857309606));
#46159=CARTESIAN_POINT('Ctrl Pts',(12.0974531385508,1.2467985598852,6.59582966877859));
#46160=CARTESIAN_POINT('Ctrl Pts',(11.9396509996858,-2.1662321888693,7.09305652013331));
#46161=CARTESIAN_POINT('Ctrl Pts',(11.7818488608208,-3.61854179246299,10.2214443230196));
#46162=CARTESIAN_POINT('Ctrl Pts',(11.6240467219557,-1.7956016590295,13.1493962879665));
#46163=CARTESIAN_POINT('Ctrl Pts',(11.4662445830908,1.65259091012735,13.2267360548792));
#46164=CARTESIAN_POINT('Ctrl Pts',(11.3084424442257,3.60497432328288,10.3834611087496));
#46165=CARTESIAN_POINT('Ctrl Pts',(11.1506403053608,2.29438831935563,7.19310410595708));
#46166=CARTESIAN_POINT('Ctrl Pts',(10.9928381664957,-1.09291675350356,6.5433520284504));
#46167=CARTESIAN_POINT('Ctrl Pts',(10.8350360276307,-3.49099038466235,9.02231474579732));
#46168=CARTESIAN_POINT('Ctrl Pts',(10.6772338887657,-2.72926485187264,12.3862095111631));
#46169=CARTESIAN_POINT('Ctrl Pts',(10.5194317499007,0.502799430185017,13.5902749971079));
#46170=CARTESIAN_POINT('Ctrl Pts',(10.3616296110357,3.27976499314249,11.5446760958796));
#46171=CARTESIAN_POINT('Ctrl Pts',(10.2038274721707,3.08811778788391,8.10094449581088));
#46172=CARTESIAN_POINT('Ctrl Pts',(10.0460253333057,0.101323344801963,6.37610534685446));
#46173=CARTESIAN_POINT('Ctrl Pts',(9.88822319444067,-2.97718180384226,7.93135930212979));
#46174=CARTESIAN_POINT('Ctrl Pts',(9.73042105557568,-3.36095133188827,11.3590046522174));
#46175=CARTESIAN_POINT('Ctrl Pts',(9.57261891671066,-0.702623662064588,
13.5565683145601));
#46176=CARTESIAN_POINT('Ctrl Pts',(9.41481677784566,2.59166910069841,12.5349881811848));
#46177=CARTESIAN_POINT('Ctrl Pts',(9.25701463898065,3.54016602667422,9.21889196466343));
#46178=CARTESIAN_POINT('Ctrl Pts',(9.09921250011564,1.28435171110455,6.60984400954655));
#46179=CARTESIAN_POINT('Ctrl Pts',(8.94141036125063,-2.13396416447173,7.0692419593061));
#46180=CARTESIAN_POINT('Ctrl Pts',(8.78360822238564,-3.62077209706865,10.1815199452736));
#46181=CARTESIAN_POINT('Ctrl Pts',(8.62580608352061,-1.83029914535168,13.1291833116438));
#46182=CARTESIAN_POINT('Ctrl Pts',(8.46800394465562,1.61680800983869,13.245137596954));
#46183=CARTESIAN_POINT('Ctrl Pts',(8.31020180579059,3.60054044813756,10.4226504132617));
#46184=CARTESIAN_POINT('Ctrl Pts',(8.15239966692561,2.32522637585507,7.21986911759536));
#46185=CARTESIAN_POINT('Ctrl Pts',(7.99459752806058,-1.05453388826692,6.52907745913553));
#46186=CARTESIAN_POINT('Ctrl Pts',(7.83679538919558,-3.48026767237864,8.9887322426102));
#46187=CARTESIAN_POINT('Ctrl Pts',(7.73159396328557,-2.99617087576157,11.2252327859881));
#46188=CARTESIAN_POINT('Ctrl Pts',(7.67899325033057,-2.33606265769622,11.9973015569306));
#46189=CARTESIAN_POINT('Ctrl Pts',(25.9332414696963,-2.81993930255816,9.37594148965641));
#46190=CARTESIAN_POINT('Ctrl Pts',(25.8806407567413,-3.02619065694277,10.3079315046869));
#46191=CARTESIAN_POINT('Ctrl Pts',(25.7754393308313,-2.43933177044069,12.3766075622725));
#46192=CARTESIAN_POINT('Ctrl Pts',(25.6176371919662,0.659289653036446,13.3444735591669));
#46193=CARTESIAN_POINT('Ctrl Pts',(25.4598350531013,3.15689027586569,11.2780546690366));
#46194=CARTESIAN_POINT('Ctrl Pts',(25.3020329142362,2.79918909152747,8.05838883695592));
#46195=CARTESIAN_POINT('Ctrl Pts',(25.1442307753712,-0.0932146705834936,
6.59429920647375));
#46196=CARTESIAN_POINT('Ctrl Pts',(24.9864286365063,-2.90069123054593,8.21376124529306));
#46197=CARTESIAN_POINT('Ctrl Pts',(24.8286264976412,-3.08295437234279,11.449507652376));
#46198=CARTESIAN_POINT('Ctrl Pts',(24.6708243587762,-0.474594130028695,
13.3735177678079));
#46199=CARTESIAN_POINT('Ctrl Pts',(24.5130222199112,2.56325762226307,12.2439236712431));
#46200=CARTESIAN_POINT('Ctrl Pts',(24.3552200810462,3.28106907303217,9.0833566147961));
#46201=CARTESIAN_POINT('Ctrl Pts',(24.1974179421812,1.02906641886227,6.75243487971409));
#46202=CARTESIAN_POINT('Ctrl Pts',(24.0396158033162,-2.15436395867484,7.36099948382184));
#46203=CARTESIAN_POINT('Ctrl Pts',(23.8818136644512,-3.38782112856686,10.3581922339581));
#46204=CARTESIAN_POINT('Ctrl Pts',(23.7240115255861,-1.55485775915207,13.0311795640836));
#46205=CARTESIAN_POINT('Ctrl Pts',(23.5662093867212,1.68545206306958,12.9605535638652));
#46206=CARTESIAN_POINT('Ctrl Pts',(23.4084072478561,3.40020991387353,10.2102438836502));
#46207=CARTESIAN_POINT('Ctrl Pts',(23.2506051089912,2.03733629025491,7.26963551251533));
#46208=CARTESIAN_POINT('Ctrl Pts',(23.0928029701261,-1.16959075609135,6.80036156342144));
#46209=CARTESIAN_POINT('Ctrl Pts',(22.9350008312611,-3.31788655382721,9.22717528280597));
#46210=CARTESIAN_POINT('Ctrl Pts',(22.7771986923961,-2.46306455045614,12.3534957241472));
#46211=CARTESIAN_POINT('Ctrl Pts',(22.6193965535311,0.621150361994919,13.3495971771476));
#46212=CARTESIAN_POINT('Ctrl Pts',(22.4615944146661,3.1431436336748,11.3138786852401));
#46213=CARTESIAN_POINT('Ctrl Pts',(22.3037922758011,2.8201841649086,8.08892952667795));
#46214=CARTESIAN_POINT('Ctrl Pts',(22.1459901369361,-0.0554078169742211,
6.59374706700197));
#46215=CARTESIAN_POINT('Ctrl Pts',(21.988187998071,-2.88084853889101,8.18166538373033));
#46216=CARTESIAN_POINT('Ctrl Pts',(21.8303858592061,-3.09874761425726,11.4154124133468));
#46217=CARTESIAN_POINT('Ctrl Pts',(21.672583720341,-0.511878114645344,13.3680275936803));
#46218=CARTESIAN_POINT('Ctrl Pts',(21.5147815814761,2.5383074823506,12.2721408852797));
#46219=CARTESIAN_POINT('Ctrl Pts',(21.356979442611,3.29099552603032,9.11967192222973));
#46220=CARTESIAN_POINT('Ctrl Pts',(21.199177303746,1.06490569473753,6.76401407015525));
#46221=CARTESIAN_POINT('Ctrl Pts',(21.041375164881,-2.12506193509776,7.3373432724013));
#46222=CARTESIAN_POINT('Ctrl Pts',(20.883573026016,-3.39157284024481,10.3207222259841));
#46223=CARTESIAN_POINT('Ctrl Pts',(20.725770887151,-1.58827035360494,13.0138059593797));
#46224=CARTESIAN_POINT('Ctrl Pts',(20.567968748286,1.65262284123301,12.979004333933));
#46225=CARTESIAN_POINT('Ctrl Pts',(20.410166609421,3.39767797845365,10.2478173352944));
#46226=CARTESIAN_POINT('Ctrl Pts',(20.252364470556,2.0673937818102,7.29232350014334));
#46227=CARTESIAN_POINT('Ctrl Pts',(20.094562331691,-1.1341499797808,6.78762815036774));
#46228=CARTESIAN_POINT('Ctrl Pts',(19.936760192826,-3.30914088220069,9.1905460490601));
#46229=CARTESIAN_POINT('Ctrl Pts',(19.778958053961,-2.48893000832816,12.3261247796686));
#46230=CARTESIAN_POINT('Ctrl Pts',(19.621155915096,0.584085399226014,13.3562588284213));
#46231=CARTESIAN_POINT('Ctrl Pts',(19.4633537762309,3.12842775007275,11.3485432471817));
#46232=CARTESIAN_POINT('Ctrl Pts',(19.305551637366,2.84113715219189,8.12022108763298));
#46233=CARTESIAN_POINT('Ctrl Pts',(19.1477494985009,-0.0177511345963581,
6.59334269786856));
#46234=CARTESIAN_POINT('Ctrl Pts',(18.9899473596359,-2.86057234181109,8.14993109473996));
#46235=CARTESIAN_POINT('Ctrl Pts',(18.8321452207709,-3.11420449228548,11.3810718508368));
#46236=CARTESIAN_POINT('Ctrl Pts',(18.6743430819059,-0.549077587440111,
13.3621634225474));
#46237=CARTESIAN_POINT('Ctrl Pts',(18.5165409430409,2.51303576306224,12.300060940609));
#46238=CARTESIAN_POINT('Ctrl Pts',(18.3587388041759,3.3005257447326,9.15610493229186));
#46239=CARTESIAN_POINT('Ctrl Pts',(18.2009366653109,1.1006117671166,6.77598343443628));
#46240=CARTESIAN_POINT('Ctrl Pts',(18.0431345264459,-2.09549863646839,7.31401516357522));
#46241=CARTESIAN_POINT('Ctrl Pts',(17.8853323875809,-3.39491093574213,10.2832116087369));
#46242=CARTESIAN_POINT('Ctrl Pts',(17.7275302487159,-1.62148843375838,12.9960648084));
#46243=CARTESIAN_POINT('Ctrl Pts',(17.5697281098509,1.61959144816781,12.9970906923159));
#46244=CARTESIAN_POINT('Ctrl Pts',(17.4119259709859,3.39473096819725,10.2853607024581));
#46245=CARTESIAN_POINT('Ctrl Pts',(17.2541238321208,2.09719858094359,7.31534225849308));
#46246=CARTESIAN_POINT('Ctrl Pts',(17.0963216932558,-1.09857058089647,6.7752873374929));
#46247=CARTESIAN_POINT('Ctrl Pts',(16.9385195543908,-3.29999085508938,9.15401570152206));
#46248=CARTESIAN_POINT('Ctrl Pts',(16.7807174155258,-2.51449131451156,12.2984696008846));
#46249=CARTESIAN_POINT('Ctrl Pts',(16.6229152766608,0.546949057781108,13.3625103427554));
#46250=CARTESIAN_POINT('Ctrl Pts',(16.4651131377958,3.11332957988147,11.3830430231847));
#46251=CARTESIAN_POINT('Ctrl Pts',(16.3073109989308,2.86174295588559,8.1517423525428));
#46252=CARTESIAN_POINT('Ctrl Pts',(16.1495088600658,0.0199077175541609,
6.59335461784961));
#46253=CARTESIAN_POINT('Ctrl Pts',(15.9917067212008,-2.83994658769004,8.118422880663));
#46254=CARTESIAN_POINT('Ctrl Pts',(15.8339045823358,-3.12928081934688,11.3465625238408));
#46255=CARTESIAN_POINT('Ctrl Pts',(15.6761024434708,-0.586209963918693,
13.355888400282));
#46256=CARTESIAN_POINT('Ctrl Pts',(15.5183003046057,2.48745695487264,12.3276999322508));
#46257=CARTESIAN_POINT('Ctrl Pts',(15.3604981657408,3.30965264445138,9.19264106494028));
#46258=CARTESIAN_POINT('Ctrl Pts',(15.2026960268757,1.1361833465123,6.78834676839902));
#46259=CARTESIAN_POINT('Ctrl Pts',(15.0448938880107,-2.06567927126773,7.29101527778403));
#46260=CARTESIAN_POINT('Ctrl Pts',(14.8870917491457,-3.39783417855664,10.2456663834901));
#46261=CARTESIAN_POINT('Ctrl Pts',(14.7292896102807,-1.65450837062362,12.9779575430958));
#46262=CARTESIAN_POINT('Ctrl Pts',(14.5714874714157,1.58636214362221,13.0148108110173));
#46263=CARTESIAN_POINT('Ctrl Pts',(14.4136853325507,3.39136912725257,10.3228691990001));
#46264=CARTESIAN_POINT('Ctrl Pts',(14.2558831936857,2.12674710576918,7.33868907771994));
#46265=CARTESIAN_POINT('Ctrl Pts',(14.0980810548207,-1.06285693844658,6.76334057934094));
#46266=CARTESIAN_POINT('Ctrl Pts',(13.9402789159557,-3.2904375743803,9.11758873191071));
#46267=CARTESIAN_POINT('Ctrl Pts',(13.7824767770907,-2.53974535388318,12.2705335527961));
#46268=CARTESIAN_POINT('Ctrl Pts',(13.6246746382257,0.509745880037291,13.3683509637108));
#46269=CARTESIAN_POINT('Ctrl Pts',(13.4668724993607,3.09785096580137,11.4173737935446));
#46270=CARTESIAN_POINT('Ctrl Pts',(13.3090703604957,2.88199905917298,8.18348947157818));
#46271=CARTESIAN_POINT('Ctrl Pts',(13.1512682216306,0.0575641370135216,
6.59378282443903));
#46272=CARTESIAN_POINT('Ctrl Pts',(12.9934660827657,-2.81897379664414,8.08714459230016));
#46273=CARTESIAN_POINT('Ctrl Pts',(12.8356639439006,-3.1439747533033,11.3118886490544));
#46274=CARTESIAN_POINT('Ctrl Pts',(12.6778618050356,-0.623270706478959,
13.3492032938407));
#46275=CARTESIAN_POINT('Ctrl Pts',(12.5200596661706,2.46157418342764,12.3550544826649));
#46276=CARTESIAN_POINT('Ctrl Pts',(12.3622575273056,3.31837510991545,9.22927585560335));
#46277=CARTESIAN_POINT('Ctrl Pts',(12.2044553884406,1.17161608612606,6.80110256115527));
#46278=CARTESIAN_POINT('Ctrl Pts',(12.0466532495756,-2.03560748337488,7.26834642575728));
#46279=CARTESIAN_POINT('Ctrl Pts',(11.8888511107106,-3.40034221146311,10.2080911378779));
#46280=CARTESIAN_POINT('Ctrl Pts',(11.7310489718456,-1.6873261292404,12.9594863767785));
#46281=CARTESIAN_POINT('Ctrl Pts',(11.5732468329806,1.55293898821088,13.0321625234532));
#46282=CARTESIAN_POINT('Ctrl Pts',(11.4154446941155,3.38759286633963,10.3603382437786));
#46283=CARTESIAN_POINT('Ctrl Pts',(11.2576425552506,2.15603574568156,7.36236110038124));
#46284=CARTESIAN_POINT('Ctrl Pts',(11.0998404163855,-1.02701341692224,6.75178934445078));
#46285=CARTESIAN_POINT('Ctrl Pts',(10.9420382775205,-3.28048220681167,9.08126957485612));
#46286=CARTESIAN_POINT('Ctrl Pts',(10.7842361386555,-2.56468904170603,12.2423200812833));
#46287=CARTESIAN_POINT('Ctrl Pts',(10.6264339997905,0.472480414602034,13.3737799156707));
#46288=CARTESIAN_POINT('Ctrl Pts',(10.4686318609255,3.08199379459717,11.4515314823219));
#46289=CARTESIAN_POINT('Ctrl Pts',(10.3108297220605,2.90190299583755,8.21545833566004));
#46290=CARTESIAN_POINT('Ctrl Pts',(10.1530275831955,0.0952135048030617,
6.59462770758856));
#46291=CARTESIAN_POINT('Ctrl Pts',(9.99522544433049,-2.79765649795469,8.05609919996786));
#46292=CARTESIAN_POINT('Ctrl Pts',(9.83742330546549,-3.15828456321738,11.2770561042392));
#46293=CARTESIAN_POINT('Ctrl Pts',(9.67962116660047,-0.660255161863091,
13.3421057601546));
#46294=CARTESIAN_POINT('Ctrl Pts',(9.52181902773547,2.43539037178042,12.3821273353805));
#46295=CARTESIAN_POINT('Ctrl Pts',(9.36401688887045,3.32669253707703,9.26599310534422));
#46296=CARTESIAN_POINT('Ctrl Pts',(9.20621475000546,1.20690476664664,6.81427183132325));
#46297=CARTESIAN_POINT('Ctrl Pts',(9.04841261114043,-2.00528523432192,7.24596789289169));
#46298=CARTESIAN_POINT('Ctrl Pts',(8.89061047227545,-3.40243802776979,10.1705742167804));
#46299=CARTESIAN_POINT('Ctrl Pts',(8.73280833341042,-1.71993134264949,12.940492251368));
#46300=CARTESIAN_POINT('Ctrl Pts',(8.57500619454543,1.5193138117507,13.0494544448574));
#46301=CARTESIAN_POINT('Ctrl Pts',(8.41720405568041,3.38342635571692,10.3971644168652));
#46302=CARTESIAN_POINT('Ctrl Pts',(8.25940191681541,2.18501425449772,7.38751217064205));
#46303=CARTESIAN_POINT('Ctrl Pts',(8.10159977795039,-0.990945054486066,
6.73837553762593));
#46304=CARTESIAN_POINT('Ctrl Pts',(7.94379763908539,-3.27040607855591,9.04971211063347));
#46305=CARTESIAN_POINT('Ctrl Pts',(7.83859621317538,-2.81550052090843,11.1513507373997));
#46306=CARTESIAN_POINT('Ctrl Pts',(7.78599550022038,-2.19519710401918,11.8768634390787));
#46307=CARTESIAN_POINT('Ctrl Pts',(26.0402437195861,-2.63898411158091,9.41598725476127));
#46308=CARTESIAN_POINT('Ctrl Pts',(25.9876430066311,-2.8320003395257,10.2881715743267));
#46309=CARTESIAN_POINT('Ctrl Pts',(25.8824415807211,-2.28280012240964,12.2241009196938));
#46310=CARTESIAN_POINT('Ctrl Pts',(25.724639441856,0.61698310942882,13.1298590633625));
#46311=CARTESIAN_POINT('Ctrl Pts',(25.5668373029911,2.95431297845888,11.1960420432666));
#46312=CARTESIAN_POINT('Ctrl Pts',(25.409035164126,2.61956543928103,8.18298180904346));
#46313=CARTESIAN_POINT('Ctrl Pts',(25.251233025261,-0.0872330955538401,
6.81284264708782));
#46314=CARTESIAN_POINT('Ctrl Pts',(25.093430886396,-2.71455419734337,8.32838398724206));
#46315=CARTESIAN_POINT('Ctrl Pts',(24.935628747531,-2.88512153363051,11.3564929077605));
#46316=CARTESIAN_POINT('Ctrl Pts',(24.777826608666,-0.4441394775622,13.1570395083698));
#46317=CARTESIAN_POINT('Ctrl Pts',(24.620024469801,2.3987736661227,12.0999313391742));
#46318=CARTESIAN_POINT('Ctrl Pts',(24.462222330936,3.07052323604148,9.14217751873442));
#46319=CARTESIAN_POINT('Ctrl Pts',(24.304420192071,0.963031341375119,6.96083077178851));
#46320=CARTESIAN_POINT('Ctrl Pts',(24.146618053206,-2.0161186633868,7.53034385302897));
#46321=CARTESIAN_POINT('Ctrl Pts',(23.988815914341,-3.1704250240619,10.3352070781982));
#46322=CARTESIAN_POINT('Ctrl Pts',(23.8310137754759,-1.45508270991801,12.836669109051));
#46323=CARTESIAN_POINT('Ctrl Pts',(23.673211636611,1.57729679189794,12.7705751714006));
#46324=CARTESIAN_POINT('Ctrl Pts',(23.5154094977459,3.18201882239524,10.1967525570521));
#46325=CARTESIAN_POINT('Ctrl Pts',(23.357607358881,1.90660064741554,7.44484269758562));
#46326=CARTESIAN_POINT('Ctrl Pts',(23.1998052200159,-1.09453824753496,7.00568200554017));
#46327=CARTESIAN_POINT('Ctrl Pts',(23.0420030811509,-3.10497814319441,9.27676735883572));
#46328=CARTESIAN_POINT('Ctrl Pts',(22.8842009422859,-2.30500997257471,12.2024721656469));
#46329=CARTESIAN_POINT('Ctrl Pts',(22.7263988034209,0.581291212445702,13.1346538993481));
#46330=CARTESIAN_POINT('Ctrl Pts',(22.5685966645559,2.94144845676636,11.2295672363402));
#46331=CARTESIAN_POINT('Ctrl Pts',(22.4107945256909,2.63921326114159,8.21156270610747));
#46332=CARTESIAN_POINT('Ctrl Pts',(22.2529923868259,-0.0518523035299743,
6.81232593834445));
#46333=CARTESIAN_POINT('Ctrl Pts',(22.0951902479609,-2.69598480900199,8.29834771354115));
#46334=CARTESIAN_POINT('Ctrl Pts',(21.9373881090959,-2.89990132497028,11.3245855564225));
#46335=CARTESIAN_POINT('Ctrl Pts',(21.7795859702309,-0.479030953038463,
13.1519016381045));
#46336=CARTESIAN_POINT('Ctrl Pts',(21.6217838313659,2.37542457390961,12.1263378577287));
#46337=CARTESIAN_POINT('Ctrl Pts',(21.4639816925008,3.07981270965628,9.17616247693458));
#46338=CARTESIAN_POINT('Ctrl Pts',(21.3061795536359,0.996570814909022,6.97166692686871));
#46339=CARTESIAN_POINT('Ctrl Pts',(21.1483774147708,-1.98869694739918,7.50820565806059));
#46340=CARTESIAN_POINT('Ctrl Pts',(20.9905752759058,-3.17393598881932,10.3001415164628));
#46341=CARTESIAN_POINT('Ctrl Pts',(20.8327731370408,-1.48635122190613,12.8204103666259));
#46342=CARTESIAN_POINT('Ctrl Pts',(20.6749709981758,1.5465742175703,12.7878419576081));
#46343=CARTESIAN_POINT('Ctrl Pts',(20.5171688593108,3.17964936098926,10.231914924489));
#46344=CARTESIAN_POINT('Ctrl Pts',(20.3593667204458,1.93472935308535,7.46607479957437));
#46345=CARTESIAN_POINT('Ctrl Pts',(20.2015645815808,-1.06137170189308,6.99376569418397));
#46346=CARTESIAN_POINT('Ctrl Pts',(20.0437624427158,-3.09679368034212,9.24248861893978));
#46347=CARTESIAN_POINT('Ctrl Pts',(19.8859603038508,-2.32921564689582,12.1768576116271));
#46348=CARTESIAN_POINT('Ctrl Pts',(19.7281581649858,0.546604704209606,13.1408880732015));
#46349=CARTESIAN_POINT('Ctrl Pts',(19.5703560261207,2.92767688977609,11.2620073772027));
#46350=CARTESIAN_POINT('Ctrl Pts',(19.4125538872558,2.65882169756453,8.24084629108108));
#46351=CARTESIAN_POINT('Ctrl Pts',(19.2547517483908,-0.0166120462663256,
6.8119475175333));
#46352=CARTESIAN_POINT('Ctrl Pts',(19.0969496095257,-2.67700973323045,8.26864981034091));
#46353=CARTESIAN_POINT('Ctrl Pts',(18.9391474706607,-2.91436633685692,11.2924486239841));
#46354=CARTESIAN_POINT('Ctrl Pts',(18.7813453317957,-0.513843339807043,
13.1464137701801));
#46355=CARTESIAN_POINT('Ctrl Pts',(18.6235431929307,2.35177453803337,12.1524662862171));
#46356=CARTESIAN_POINT('Ctrl Pts',(18.4657410540657,3.08873137528585,9.21025758479872));
#46357=CARTESIAN_POINT('Ctrl Pts',(18.3079389152007,1.02998563260026,6.9828682183769));
#46358=CARTESIAN_POINT('Ctrl Pts',(18.1501367763357,-1.96103072235028,7.48637451137971));
#46359=CARTESIAN_POINT('Ctrl Pts',(17.9923346374707,-3.17705987910036,10.2650379513466));
#46360=CARTESIAN_POINT('Ctrl Pts',(17.8345324986057,-1.51743770155576,12.8038076633286));
#46361=CARTESIAN_POINT('Ctrl Pts',(17.6767303597407,1.51566244531925,12.8047677163879));
#46362=CARTESIAN_POINT('Ctrl Pts',(17.5189282208757,3.17689146005279,10.2670491379631));
#46363=CARTESIAN_POINT('Ctrl Pts',(17.3611260820106,1.96262158157783,7.48761644676452));
#46364=CARTESIAN_POINT('Ctrl Pts',(17.2033239431456,-1.02807542907254,6.98221678989685));
#46365=CARTESIAN_POINT('Ctrl Pts',(17.0455218042806,-3.08823080945147,9.20830241973473));
#46366=CARTESIAN_POINT('Ctrl Pts',(16.8877196654156,-2.3531366869083,12.1509770625856));
#46367=CARTESIAN_POINT('Ctrl Pts',(16.7299175265506,0.511851397659197,13.146738428557));
#46368=CARTESIAN_POINT('Ctrl Pts',(16.5721153876856,2.91354756748443,11.294293306422));
#46369=CARTESIAN_POINT('Ctrl Pts',(16.4143132488206,2.67810522913017,8.2703448399323));
#46370=CARTESIAN_POINT('Ctrl Pts',(16.2565111099556,0.0186302415359106,
6.81195867261049));
#46371=CARTESIAN_POINT('Ctrl Pts',(16.0987089710906,-2.65770753145417,8.23916347485209));
#46372=CARTESIAN_POINT('Ctrl Pts',(15.9409068322256,-2.92847521768991,11.260153756658));
#46373=CARTESIAN_POINT('Ctrl Pts',(15.7831046933606,-0.548592935822577,
13.1405414153946));
#46374=CARTESIAN_POINT('Ctrl Pts',(15.6253025544956,2.32783711911649,12.1783316868435));
#46375=CARTESIAN_POINT('Ctrl Pts',(15.4675004156306,3.09727260286618,9.24444919788427));
#46376=CARTESIAN_POINT('Ctrl Pts',(15.3096982767655,1.06327458770789,6.9944381985762));
#46377=CARTESIAN_POINT('Ctrl Pts',(15.1518961379006,-1.93312486249343,7.46485052569816));
#46378=CARTESIAN_POINT('Ctrl Pts',(14.9940939990355,-3.17979553774904,10.2299019990224));
#46379=CARTESIAN_POINT('Ctrl Pts',(14.8362918601705,-1.54833875274991,12.7868623392224));
#46380=CARTESIAN_POINT('Ctrl Pts',(14.6784897213055,1.48456546154546,12.8213507370459));
#46381=CARTESIAN_POINT('Ctrl Pts',(14.5206875824405,3.17374534806711,10.3021507184595));
#46382=CARTESIAN_POINT('Ctrl Pts',(14.3628854435755,1.9902739808563,7.50946510320182));
#46383=CARTESIAN_POINT('Ctrl Pts',(14.2050833047105,-0.994653527081089,
6.97103665388494));
#46384=CARTESIAN_POINT('Ctrl Pts',(14.0472811658455,-3.0792905617015,9.17421296470632));
#46385=CARTESIAN_POINT('Ctrl Pts',(13.8894790269805,-2.37677017738608,12.1248336675916));
#46386=CARTESIAN_POINT('Ctrl Pts',(13.7316768881155,0.477035543687735,13.1522042575162));
#46387=CARTESIAN_POINT('Ctrl Pts',(13.5738747492505,2.89906221434594,11.3264210750714));
#46388=CARTESIAN_POINT('Ctrl Pts',(13.4160726103855,2.69706150052561,8.30005474987497));
#46389=CARTESIAN_POINT('Ctrl Pts',(13.2582704715205,0.0538702527525129,
6.81235940123075));
#46390=CARTESIAN_POINT('Ctrl Pts',(13.1004683326554,-2.63808056207387,8.20989231076991));
#46391=CARTESIAN_POINT('Ctrl Pts',(12.9426661937904,-2.94222624354086,11.2277049005549));
#46392=CARTESIAN_POINT('Ctrl Pts',(12.7848640549254,-0.583275494660355,
13.1342852914891));
#46393=CARTESIAN_POINT('Ctrl Pts',(12.6270619160604,2.30361524223244,12.2039308988041));
#46394=CARTESIAN_POINT('Ctrl Pts',(12.4692597771954,3.10543534869288,9.27873313811066));
#46395=CARTESIAN_POINT('Ctrl Pts',(12.3114576383304,1.09643361236692,7.00637545353194));
#46396=CARTESIAN_POINT('Ctrl Pts',(12.1536554994654,-1.90498277788045,7.44363633138125));
#46397=CARTESIAN_POINT('Ctrl Pts',(11.9958533606004,-3.18214263046322,10.1947379527362));
#46398=CARTESIAN_POINT('Ctrl Pts',(11.8380512217354,-1.5790505994513,12.7695764655905));
#46399=CARTESIAN_POINT('Ctrl Pts',(11.6802490828704,1.45328706629441,12.8375889920273));
#46400=CARTESIAN_POINT('Ctrl Pts',(11.5224469440054,3.17021140939637,10.3372153788076));
#46401=CARTESIAN_POINT('Ctrl Pts',(11.3646448051404,2.0176831720075,7.53161809480538));
#46402=CARTESIAN_POINT('Ctrl Pts',(11.2068426662754,-0.961110080340932,
6.96022666045117));
#46403=CARTESIAN_POINT('Ctrl Pts',(11.0490405274104,-3.06997402896098,9.14022440391494));
#46404=CARTESIAN_POINT('Ctrl Pts',(10.8912383885453,-2.40011323153943,12.0984306514035));
#46405=CARTESIAN_POINT('Ctrl Pts',(10.7334362496803,0.442161399019054,13.1572848342334));
#46406=CARTESIAN_POINT('Ctrl Pts',(10.5756341108153,2.88422259605183,11.3583868687642));
#46407=CARTESIAN_POINT('Ctrl Pts',(10.4178319719503,2.71568820379119,8.32997217550921));
#46408=CARTESIAN_POINT('Ctrl Pts',(10.2600298330853,0.0891036648041555,
6.81315006832269));
#46409=CARTESIAN_POINT('Ctrl Pts',(10.1022276942203,-2.61813119206713,8.1808390978059));
#46410=CARTESIAN_POINT('Ctrl Pts',(9.9444255553553,-2.9556177945465,11.195107556261));
#46411=CARTESIAN_POINT('Ctrl Pts',(9.78662341649027,-0.61788666166159,13.1276432057492));
#46412=CARTESIAN_POINT('Ctrl Pts',(9.62882127762529,2.27911164286243,12.2292664895762));
#46413=CARTESIAN_POINT('Ctrl Pts',(9.47101913876025,3.11321904747985,9.31309424602498));
#46414=CARTESIAN_POINT('Ctrl Pts',(9.31321699989528,1.12945782218873,7.01869965309997));
#46415=CARTESIAN_POINT('Ctrl Pts',(9.15541486103024,-1.87660630417212,7.42269382647725));
#46416=CARTESIAN_POINT('Ctrl Pts',(8.99761272216525,-3.18410395847092,10.1596284882871));
#46417=CARTESIAN_POINT('Ctrl Pts',(8.83981058330023,-1.6095635399473,12.7518011910921));
#46418=CARTESIAN_POINT('Ctrl Pts',(8.68200844443524,1.42181961366271,12.8537712927609));
#46419=CARTESIAN_POINT('Ctrl Pts',(8.52420630557022,3.16631226329628,10.3716784204688));
#46420=CARTESIAN_POINT('Ctrl Pts',(8.36640416670522,2.04480213314037,7.55515522368873));
#46421=CARTESIAN_POINT('Ctrl Pts',(8.20860202784021,-0.927356220705207,
6.94767361611631));
#46422=CARTESIAN_POINT('Ctrl Pts',(8.0507998889752,-3.06054448473317,9.11069197865678));
#46423=CARTESIAN_POINT('Ctrl Pts',(7.94559846306519,-2.63483016605528,11.0774686888113));
#46424=CARTESIAN_POINT('Ctrl Pts',(7.89299775011019,-2.05433155034215,11.7564253212268));
#46425=CARTESIAN_POINT('Ctrl Pts',(26.1472459694759,-2.45802892060367,9.45603301986612));
#46426=CARTESIAN_POINT('Ctrl Pts',(26.0946452565209,-2.63781002210864,10.2684116439665));
#46427=CARTESIAN_POINT('Ctrl Pts',(25.9894438306109,-2.12626847437859,12.071594277115));
#46428=CARTESIAN_POINT('Ctrl Pts',(25.8316416917459,0.574676565821197,12.9152445675582));
#46429=CARTESIAN_POINT('Ctrl Pts',(25.6738395528808,2.75173568105207,11.1140294174966));
#46430=CARTESIAN_POINT('Ctrl Pts',(25.5160374140159,2.43994178703459,8.307574781131));
#46431=CARTESIAN_POINT('Ctrl Pts',(25.3582352751508,-0.0812515205241886,
7.0313860877019));
#46432=CARTESIAN_POINT('Ctrl Pts',(25.2004331362858,-2.52841716414082,8.44300672919104));
#46433=CARTESIAN_POINT('Ctrl Pts',(25.0426309974208,-2.68728869491822,11.263478163145));
#46434=CARTESIAN_POINT('Ctrl Pts',(24.8848288585558,-0.413684825095704,
12.9405612489317));
#46435=CARTESIAN_POINT('Ctrl Pts',(24.7270267196908,2.23428970998233,11.9559390071053));
#46436=CARTESIAN_POINT('Ctrl Pts',(24.5692245808258,2.85997739905078,9.2009984226727));
#46437=CARTESIAN_POINT('Ctrl Pts',(24.4114224419608,0.896996263887967,7.16922666386296));
#46438=CARTESIAN_POINT('Ctrl Pts',(24.2536203030958,-1.87787336809876,7.69968822223608));
#46439=CARTESIAN_POINT('Ctrl Pts',(24.0958181642307,-2.95302891955695,10.3122219224385));
#46440=CARTESIAN_POINT('Ctrl Pts',(23.9380160253658,-1.35530766068394,12.6421586540183));
#46441=CARTESIAN_POINT('Ctrl Pts',(23.7802138865008,1.4691415207263,12.5805967789361));
#46442=CARTESIAN_POINT('Ctrl Pts',(23.6224117476358,2.96382773091694,10.183261230454));
#46443=CARTESIAN_POINT('Ctrl Pts',(23.4646096087708,1.77586500457617,7.62004988265589));
#46444=CARTESIAN_POINT('Ctrl Pts',(23.3068074699057,-1.01948573897858,7.2110024476589));
#46445=CARTESIAN_POINT('Ctrl Pts',(23.1490053310407,-2.8920697325616,9.32635943486548));
#46446=CARTESIAN_POINT('Ctrl Pts',(22.9912031921758,-2.14695539469329,12.0514486071466));
#46447=CARTESIAN_POINT('Ctrl Pts',(22.8334010533107,0.541432062896488,12.9197106215485));
#46448=CARTESIAN_POINT('Ctrl Pts',(22.6755989144457,2.73975327985792,11.1452557874403));
#46449=CARTESIAN_POINT('Ctrl Pts',(22.5177967755807,2.45824235737459,8.33419588553699));
#46450=CARTESIAN_POINT('Ctrl Pts',(22.3599946367157,-0.0482967900857281,
7.03090480968693));
#46451=CARTESIAN_POINT('Ctrl Pts',(22.2021924978507,-2.51112107911298,8.41503004335198));
#46452=CARTESIAN_POINT('Ctrl Pts',(22.0443903589857,-2.7010550356833,11.2337586994981));
#46453=CARTESIAN_POINT('Ctrl Pts',(21.8865882201206,-0.446183791431585,
12.9357756825288));
#46454=CARTESIAN_POINT('Ctrl Pts',(21.7287860812557,2.21254166546862,11.9805348301777));
#46455=CARTESIAN_POINT('Ctrl Pts',(21.5709839423906,2.86862989328224,9.23265303163944));
#46456=CARTESIAN_POINT('Ctrl Pts',(21.4131818035257,0.928235935080519,7.17931978358216));
#46457=CARTESIAN_POINT('Ctrl Pts',(21.2553796646606,-1.85233195970059,7.67906804371988));
#46458=CARTESIAN_POINT('Ctrl Pts',(21.0975775257957,-2.95629913739384,10.2795608069415));
#46459=CARTESIAN_POINT('Ctrl Pts',(20.9397753869306,-1.38443209020732,12.6270147738721));
#46460=CARTESIAN_POINT('Ctrl Pts',(20.7819732480656,1.44052559390759,12.5966795812833));
#46461=CARTESIAN_POINT('Ctrl Pts',(20.6241711092006,2.96162074352487,10.2160125136836));
#46462=CARTESIAN_POINT('Ctrl Pts',(20.4663689703356,1.8020649243605,7.63982609900542));
#46463=CARTESIAN_POINT('Ctrl Pts',(20.3085668314706,-0.988593424005365,
7.19990323800016));
#46464=CARTESIAN_POINT('Ctrl Pts',(20.1507646926056,-2.88444647848355,9.29443118881948));
#46465=CARTESIAN_POINT('Ctrl Pts',(19.9929625537406,-2.16950128546349,12.0275904435855));
#46466=CARTESIAN_POINT('Ctrl Pts',(19.8351604148756,0.509124009193201,12.9255173179817));
#46467=CARTESIAN_POINT('Ctrl Pts',(19.6773582760106,2.72692602947942,11.1754715072237));
#46468=CARTESIAN_POINT('Ctrl Pts',(19.5195561371456,2.47650624293718,8.36147149452918));
#46469=CARTESIAN_POINT('Ctrl Pts',(19.3617539982806,-0.0154729579362931,
7.03055233719803));
#46470=CARTESIAN_POINT('Ctrl Pts',(19.2039518594155,-2.49344712464981,8.38736852594188));
#46471=CARTESIAN_POINT('Ctrl Pts',(19.0461497205505,-2.71452818142837,11.2038253971314));
#46472=CARTESIAN_POINT('Ctrl Pts',(18.8883475816855,-0.478609092173977,
12.9306641178128));
#46473=CARTESIAN_POINT('Ctrl Pts',(18.7305454428205,2.19051331300451,12.0048716318252));
#46474=CARTESIAN_POINT('Ctrl Pts',(18.5727433039555,2.87693700583911,9.26441023730558));
#46475=CARTESIAN_POINT('Ctrl Pts',(18.4149411650905,0.959359498083921,7.1897530023175));
#46476=CARTESIAN_POINT('Ctrl Pts',(18.2571390262255,-1.82656280823216,7.65873385918423));
#46477=CARTESIAN_POINT('Ctrl Pts',(18.0993368873605,-2.95920882245859,10.2468642939564));
#46478=CARTESIAN_POINT('Ctrl Pts',(17.9415347484955,-1.41338696935313,12.6115505182573));
#46479=CARTESIAN_POINT('Ctrl Pts',(17.7837326096305,1.4117334424707,12.61244474046));
#46480=CARTESIAN_POINT('Ctrl Pts',(17.6259304707655,2.95905195190833,10.2487375734681));
#46481=CARTESIAN_POINT('Ctrl Pts',(17.4681283319004,1.82804458221207,7.65989063503597));
#46482=CARTESIAN_POINT('Ctrl Pts',(17.3103261930355,-0.95758027724861,7.18914624230078));
#46483=CARTESIAN_POINT('Ctrl Pts',(17.1525240541704,-2.87647076381356,9.26258913794742));
#46484=CARTESIAN_POINT('Ctrl Pts',(16.9947219153054,-2.19178205930505,12.0034845242866));
#46485=CARTESIAN_POINT('Ctrl Pts',(16.8369197764404,0.476753737537289,12.9309665143586));
#46486=CARTESIAN_POINT('Ctrl Pts',(16.6791176375754,2.7137655550874,11.2055435896593));
#46487=CARTESIAN_POINT('Ctrl Pts',(16.5213154987104,2.49446750237474,8.38894732732178));
#46488=CARTESIAN_POINT('Ctrl Pts',(16.3635133598454,0.0173527655176627,
7.03056272737136));
#46489=CARTESIAN_POINT('Ctrl Pts',(16.2057112209804,-2.47546847521831,8.35990406904119));
#46490=CARTESIAN_POINT('Ctrl Pts',(16.0479090821154,-2.72766961603293,11.1737449894752));
#46491=CARTESIAN_POINT('Ctrl Pts',(15.8901069432504,-0.51097590772646,12.9251944305072));
#46492=CARTESIAN_POINT('Ctrl Pts',(15.7323048043854,2.16821728336033,12.0289634414362));
#46493=CARTESIAN_POINT('Ctrl Pts',(15.5745026655204,2.88489256128098,9.29625733082825));
#46494=CARTESIAN_POINT('Ctrl Pts',(15.4167005266553,0.990365828903469,7.20052962875338));
#46495=CARTESIAN_POINT('Ctrl Pts',(15.2588983877904,-1.80057045371914,7.63868577361231));
#46496=CARTESIAN_POINT('Ctrl Pts',(15.1010962489253,-2.96175689694143,10.2141376145547));
#46497=CARTESIAN_POINT('Ctrl Pts',(14.9432941100604,-1.44216913487621,12.595767135349));
#46498=CARTESIAN_POINT('Ctrl Pts',(14.7854919711953,1.38276877946872,12.6278906630745));
#46499=CARTESIAN_POINT('Ctrl Pts',(14.6276898323303,2.95612156888165,10.2814322379189));
#46500=CARTESIAN_POINT('Ctrl Pts',(14.4698876934653,1.85380085594341,7.6802411286837));
#46501=CARTESIAN_POINT('Ctrl Pts',(14.3120855546003,-0.926450115715597,
7.17873272842893));
#46502=CARTESIAN_POINT('Ctrl Pts',(14.1542834157353,-2.8681435490227,9.23083719750194));
#46503=CARTESIAN_POINT('Ctrl Pts',(13.9964812768703,-2.21379500088899,11.9791337823871));
#46504=CARTESIAN_POINT('Ctrl Pts',(13.8386791380053,0.444325207338179,12.9360575513216));
#46505=CARTESIAN_POINT('Ctrl Pts',(13.6808769991403,2.70027346289051,11.2354683565983));
#46506=CARTESIAN_POINT('Ctrl Pts',(13.5230748602753,2.51212394187823,8.41662002817174));
#46507=CARTESIAN_POINT('Ctrl Pts',(13.3652727214103,0.0501763684915025,
7.03093597802249));
#46508=CARTESIAN_POINT('Ctrl Pts',(13.2074705825453,-2.45718732750359,8.33264002923965));
#46509=CARTESIAN_POINT('Ctrl Pts',(13.0496684436802,-2.74047773377842,11.1435211520554));
#46510=CARTESIAN_POINT('Ctrl Pts',(12.8918663048152,-0.543280282841749,
12.9193672891375));
#46511=CARTESIAN_POINT('Ctrl Pts',(12.7340641659502,2.14565630103725,12.0528073149434));
#46512=CARTESIAN_POINT('Ctrl Pts',(12.5762620270852,2.8924955874703,9.32819042061796));
#46513=CARTESIAN_POINT('Ctrl Pts',(12.4184598882202,1.02125113860777,7.21164834590862));
#46514=CARTESIAN_POINT('Ctrl Pts',(12.2606577493552,-1.77435807238603,7.61892623700522));
#46515=CARTESIAN_POINT('Ctrl Pts',(12.1028556104902,-2.96394304946334,10.1813847675946));
#46516=CARTESIAN_POINT('Ctrl Pts',(11.9450534716252,-1.4707750696622,12.5796665544024));
#46517=CARTESIAN_POINT('Ctrl Pts',(11.7872513327602,1.35363514437794,12.6430154606013));
#46518=CARTESIAN_POINT('Ctrl Pts',(11.6294491938952,2.95282995245311,10.3140925138367));
#46519=CARTESIAN_POINT('Ctrl Pts',(11.4716470550302,1.87933059833343,7.70087508922953));
#46520=CARTESIAN_POINT('Ctrl Pts',(11.3138449161652,-0.895206743759622,
7.16866397645156));
#46521=CARTESIAN_POINT('Ctrl Pts',(11.1560427773002,-2.85946585111029,9.19917923297374));
#46522=CARTESIAN_POINT('Ctrl Pts',(10.9982406384351,-2.23553742137283,11.9545412215237));
#46523=CARTESIAN_POINT('Ctrl Pts',(10.8404384995701,0.411842383436077,12.9407897527962));
#46524=CARTESIAN_POINT('Ctrl Pts',(10.6826363607051,2.6864513975065,11.2652422552064));
#46525=CARTESIAN_POINT('Ctrl Pts',(10.5248342218401,2.52947341174483,8.44448601535835));
#46526=CARTESIAN_POINT('Ctrl Pts',(10.3670320829751,0.0829938248052507,
7.03167242905681));
#46527=CARTESIAN_POINT('Ctrl Pts',(10.2092299441101,-2.43860588617956,8.30557899564397));
#46528=CARTESIAN_POINT('Ctrl Pts',(10.0514278052451,-2.75295102587562,11.1131590082828));
#46529=CARTESIAN_POINT('Ctrl Pts',(9.8936256663801,-0.575518161460093,12.9131806513437));
#46530=CARTESIAN_POINT('Ctrl Pts',(9.73582352751509,2.12283291394444,12.0764056437719));
#46531=CARTESIAN_POINT('Ctrl Pts',(9.57802138865008,2.89974555788266,9.36019538670575));
#46532=CARTESIAN_POINT('Ctrl Pts',(9.42021924978507,1.05201087773083,7.22312747487668));
#46533=CARTESIAN_POINT('Ctrl Pts',(9.26241711092007,-1.74792737402231,7.59941976006281));
#46534=CARTESIAN_POINT('Ctrl Pts',(9.10461497205506,-2.96576988917206,10.1486827597939));
#46535=CARTESIAN_POINT('Ctrl Pts',(8.94681283319005,-1.49919573724511,12.5631101308161));
#46536=CARTESIAN_POINT('Ctrl Pts',(8.78901069432504,1.32432541557472,12.6580881406643));
#46537=CARTESIAN_POINT('Ctrl Pts',(8.63120855546003,2.94919817087565,10.3461924240723));
#46538=CARTESIAN_POINT('Ctrl Pts',(8.47340641659503,1.90459001178303,7.72279827673542));
#46539=CARTESIAN_POINT('Ctrl Pts',(8.31560427773002,-0.863767386924347,
7.1569716946067));
#46540=CARTESIAN_POINT('Ctrl Pts',(8.15780213886501,-2.85068289091044,9.17167184668006));
#46541=CARTESIAN_POINT('Ctrl Pts',(8.05260071295501,-2.45415981120213,11.0035866402229));
#46542=CARTESIAN_POINT('Ctrl Pts',(8.,-1.91346599666512,11.6359872033749));
#46543=CARTESIAN_POINT('Ctrl Pts',(25.8262392198064,-3.00089449353543,9.33589572455167));
#46544=CARTESIAN_POINT('Ctrl Pts',(25.8247009270193,-3.01413331869119,9.41774832515779));
#46545=CARTESIAN_POINT('Ctrl Pts',(25.8236428523257,-3.02293576180228,9.50001791442205));
#46546=CARTESIAN_POINT('Ctrl Pts',(25.8230736514177,-3.02740143036249,9.58247963833164));
#46547=CARTESIAN_POINT('Ctrl Pts',(25.8224963555106,-3.03193060827776,9.66611410733683));
#46548=CARTESIAN_POINT('Ctrl Pts',(25.8224219374901,-3.03199837110086,9.74994735780831));
#46549=CARTESIAN_POINT('Ctrl Pts',(25.8228594276208,-3.02765701722773,9.83373247955964));
#46550=CARTESIAN_POINT('Ctrl Pts',(25.8231188569373,-3.02508261751192,9.88341661034674));
#46551=CARTESIAN_POINT('Ctrl Pts',(25.8235582950085,-3.02095683206533,9.93308349902347));
#46552=CARTESIAN_POINT('Ctrl Pts',(25.8241796248454,-3.01528316277101,9.98267714040271));
#46553=CARTESIAN_POINT('Ctrl Pts',(25.8252586009475,-3.00543049963359,10.0687994392043));
#46554=CARTESIAN_POINT('Ctrl Pts',(25.8268799435765,-2.99097538638735,10.1541420483801));
#46555=CARTESIAN_POINT('Ctrl Pts',(25.8289948543176,-2.97214067508313,10.2384343398583));
#46556=CARTESIAN_POINT('Ctrl Pts',(25.8311660717319,-2.95280451475119,10.3249708009935));
#46557=CARTESIAN_POINT('Ctrl Pts',(25.8338574882923,-2.92885232911599,10.4104015543961));
#46558=CARTESIAN_POINT('Ctrl Pts',(25.8370163033174,-2.9004704184457,10.4944373216573));
#46559=CARTESIAN_POINT('Ctrl Pts',(25.8395515325628,-2.87769141765036,10.5618834788776));
#46560=CARTESIAN_POINT('Ctrl Pts',(25.842387835885,-2.85205786037235,10.6284313817431));
#46561=CARTESIAN_POINT('Ctrl Pts',(25.8454979160497,-2.82364278082183,10.693924553429));
#46562=CARTESIAN_POINT('Ctrl Pts',(25.8494069505495,-2.7879280981151,10.7762423890014));
#46563=CARTESIAN_POINT('Ctrl Pts',(25.8537216893179,-2.74802249289677,10.8564504017753));
#46564=CARTESIAN_POINT('Ctrl Pts',(25.8583471798576,-2.70422623397282,10.934271696085));
#46565=CARTESIAN_POINT('Ctrl Pts',(25.8630134592934,-2.66004376713455,11.0127792407847));
#46566=CARTESIAN_POINT('Ctrl Pts',(25.8679959952607,-2.61190187709947,11.0888588190426));
#46567=CARTESIAN_POINT('Ctrl Pts',(25.8731973010912,-2.56005798819279,11.1622409925269));
#46568=CARTESIAN_POINT('Ctrl Pts',(25.8783373476878,-2.50882469920387,11.2347588954087));
#46569=CARTESIAN_POINT('Ctrl Pts',(25.8836910412979,-2.45397610829872,11.3046435898681));
#46570=CARTESIAN_POINT('Ctrl Pts',(25.8891642993397,-2.39571031021884,11.3716340572743));
#46571=CARTESIAN_POINT('Ctrl Pts',(25.8901970757974,-2.38471584511528,11.3842748239066));
#46572=CARTESIAN_POINT('Ctrl Pts',(25.8912341094429,-2.37359956143892,11.3968125106867));
#46573=CARTESIAN_POINT('Ctrl Pts',(25.8922747681696,-2.36236258457764,11.409245313078));
#46574=CARTESIAN_POINT('Ctrl Pts',(25.8980643682246,-2.2998467951173,11.4784139574821));
#46575=CARTESIAN_POINT('Ctrl Pts',(25.9039451254502,-2.23378997666101,11.5441355297943));
#46576=CARTESIAN_POINT('Ctrl Pts',(25.9098076340753,-2.1644479552529,11.606113861888));
#46577=CARTESIAN_POINT('Ctrl Pts',(25.9152817910467,-2.09969937505019,11.6639865475251));
#46578=CARTESIAN_POINT('Ctrl Pts',(25.9207400370331,-2.03208631420079,11.7185964264391));
#46579=CARTESIAN_POINT('Ctrl Pts',(25.9260932999764,-1.96176778668457,11.7697004547667));
#46580=CARTESIAN_POINT('Ctrl Pts',(25.9264730750774,-1.95677919819684,11.7733259141783));
#46581=CARTESIAN_POINT('Ctrl Pts',(25.9268523218122,-1.95177697185848,11.7769337248518));
#46582=CARTESIAN_POINT('Ctrl Pts',(25.9272310083782,-1.94676115438266,11.7805237977182));
#46583=CARTESIAN_POINT('Ctrl Pts',(25.9290252763024,-1.92299553600559,11.7975340462171));
#46584=CARTESIAN_POINT('Ctrl Pts',(25.9308060613756,-1.89893491844326,11.814139212597));
#46585=CARTESIAN_POINT('Ctrl Pts',(25.9325705627918,-1.87458502252745,11.830329187418));
#46586=CARTESIAN_POINT('Ctrl Pts',(25.9384088208045,-1.79401780187663,11.8838974358511));
#46587=CARTESIAN_POINT('Ctrl Pts',(25.944068810366,-1.71028733025863,11.9329202536286));
#46588=CARTESIAN_POINT('Ctrl Pts',(25.9494490780203,-1.62397669191922,11.9774031117903));
#46589=CARTESIAN_POINT('Ctrl Pts',(25.9530493859837,-1.56622029418781,12.0071696585063));
#46590=CARTESIAN_POINT('Ctrl Pts',(25.9565244380966,-1.50730751226311,12.0349033850039));
#46591=CARTESIAN_POINT('Ctrl Pts',(25.9598438343188,-1.44740009951426,12.0606038454663));
#46592=CARTESIAN_POINT('Ctrl Pts',(8.,-1.91346599666512,11.6359872033749));
#46593=CARTESIAN_POINT('Ctrl Pts',(8.,-1.97562899072746,11.5775692532266));
#46594=CARTESIAN_POINT('Ctrl Pts',(8.00000000000001,-2.0344185889114,11.5158993410469));
#46595=CARTESIAN_POINT('Ctrl Pts',(8.00000000000001,-2.08982174948349,11.4513534699324));
#46596=CARTESIAN_POINT('Ctrl Pts',(8.00000000000001,-2.1465762488304,11.3852332601432));
#46597=CARTESIAN_POINT('Ctrl Pts',(8.00000000000001,-2.19977756879385,11.316094593968));
#46598=CARTESIAN_POINT('Ctrl Pts',(8.00000000000001,-2.24938282561102,11.2442953918663));
#46599=CARTESIAN_POINT('Ctrl Pts',(8.00000000000001,-2.26237822312376,11.2254857085327));
#46600=CARTESIAN_POINT('Ctrl Pts',(8.,-2.27512664525496,11.2064932102818));
#46601=CARTESIAN_POINT('Ctrl Pts',(8.,-2.28762694073546,11.1873238938734));
#46602=CARTESIAN_POINT('Ctrl Pts',(8.,-2.2977159200289,11.1718523526915));
#46603=CARTESIAN_POINT('Ctrl Pts',(8.00000000000001,-2.30764363777327,11.1562648370275));
#46604=CARTESIAN_POINT('Ctrl Pts',(8.00000000000001,-2.31740083565843,11.1405787745481));
#46605=CARTESIAN_POINT('Ctrl Pts',(8.00000000000001,-2.36487425058001,11.0642586095444));
#46606=CARTESIAN_POINT('Ctrl Pts',(8.,-2.40836451010314,10.9855325134811));
#46607=CARTESIAN_POINT('Ctrl Pts',(8.,-2.44783576857742,10.9047923278186));
#46608=CARTESIAN_POINT('Ctrl Pts',(8.,-2.47963039280521,10.8397550332795));
#46609=CARTESIAN_POINT('Ctrl Pts',(8.00000000000001,-2.50881677888913,10.7734098051544));
#46610=CARTESIAN_POINT('Ctrl Pts',(8.00000000000001,-2.53535914135491,10.7059437471017));
#46611=CARTESIAN_POINT('Ctrl Pts',(8.00000000000001,-2.5456178511057,10.6798678953954));
#46612=CARTESIAN_POINT('Ctrl Pts',(8.,-2.55548141093818,10.6536244660234));
#46613=CARTESIAN_POINT('Ctrl Pts',(8.,-2.56494707540061,10.6272237735826));
#46614=CARTESIAN_POINT('Ctrl Pts',(8.,-2.57037504020302,10.6120846325433));
#46615=CARTESIAN_POINT('Ctrl Pts',(8.00000000000001,-2.57567218840733,10.5968934250601));
#46616=CARTESIAN_POINT('Ctrl Pts',(8.00000000000001,-2.58083326929062,10.5816666265579));
#46617=CARTESIAN_POINT('Ctrl Pts',(8.00000000000001,-2.61045215866775,10.4942816638723));
#46618=CARTESIAN_POINT('Ctrl Pts',(8.00000000000001,-2.63563451227559,10.4056131148661));
#46619=CARTESIAN_POINT('Ctrl Pts',(8.00000000000001,-2.65634683466178,10.3160581348443));
#46620=CARTESIAN_POINT('Ctrl Pts',(8.00000000000001,-2.6773791473997,10.2251195953634));
#46621=CARTESIAN_POINT('Ctrl Pts',(8.00000000000001,-2.6938027464082,10.133266219799));
#46622=CARTESIAN_POINT('Ctrl Pts',(8.00000000000001,-2.70554079647472,10.0408806216262));
#46623=CARTESIAN_POINT('Ctrl Pts',(8.00000000000001,-2.71718716742871,9.94921659386775));
#46624=CARTESIAN_POINT('Ctrl Pts',(8.00000000000001,-2.72422124186341,9.85702769697448));
#46625=CARTESIAN_POINT('Ctrl Pts',(8.00000000000001,-2.726521063454,9.76466836326314));
#46626=CARTESIAN_POINT('Ctrl Pts',(8.00000000000001,-2.72766371249266,9.71878032381365));
#46627=CARTESIAN_POINT('Ctrl Pts',(8.,-2.72763693803085,9.67284999779573));
#46628=CARTESIAN_POINT('Ctrl Pts',(8.,-2.72642101212846,9.62692015028946));
#46629=CARTESIAN_POINT('Ctrl Pts',(8.,-2.72605450623643,9.61307591874715));
#46630=CARTESIAN_POINT('Ctrl Pts',(8.00000000000001,-2.72557993734327,9.59923172991306));
#46631=CARTESIAN_POINT('Ctrl Pts',(8.00000000000001,-2.72499670497433,9.58538875478852));
#46632=CARTESIAN_POINT('Ctrl Pts',(8.00000000000001,-2.72437261249071,9.57057596800533));
#46633=CARTESIAN_POINT('Ctrl Pts',(8.00000000000001,-2.72362445980719,9.5557737118897));
#46634=CARTESIAN_POINT('Ctrl Pts',(8.00000000000001,-2.72275224759148,9.54098749246186));
#46635=CARTESIAN_POINT('Ctrl Pts',(8.,-2.71711692851713,9.44545447552171));
#46636=CARTESIAN_POINT('Ctrl Pts',(8.,-2.70630452088264,9.3505388335816));
#46637=CARTESIAN_POINT('Ctrl Pts',(8.,-2.69024345035316,9.25663514051171));
#46638=CARTESIAN_POINT('Ctrl Pts',(8.,-2.68799188729149,9.24347100638487));
#46639=CARTESIAN_POINT('Ctrl Pts',(8.00000000000001,-2.68563709640445,9.23032672963803));
#46640=CARTESIAN_POINT('Ctrl Pts',(8.00000000000001,-2.68317880266814,9.21720337142564));
#46641=CARTESIAN_POINT('Ctrl Pts',(8.00000000000001,-2.66632395667961,9.12722544150852));
#46642=CARTESIAN_POINT('Ctrl Pts',(8.,-2.64460792115915,9.03823106363511));
#46643=CARTESIAN_POINT('Ctrl Pts',(8.,-2.6183336817708,8.95045339427309));
#46644=CARTESIAN_POINT('Ctrl Pts',(8.,-2.59146203306373,8.86067988416082));
#46645=CARTESIAN_POINT('Ctrl Pts',(8.00000000000001,-2.55982233228106,8.77217834086338));
#46646=CARTESIAN_POINT('Ctrl Pts',(8.00000000000001,-2.52368444078896,8.68520171010531));
#46647=CARTESIAN_POINT('Ctrl Pts',(8.00000000000001,-2.51182298835605,8.65665358164747));
#46648=CARTESIAN_POINT('Ctrl Pts',(8.00000000000001,-2.49947651817337,8.62826981102031));
#46649=CARTESIAN_POINT('Ctrl Pts',(8.00000000000001,-2.48665340280304,8.60005962686124));
#46650=CARTESIAN_POINT('Ctrl Pts',(8.00000000000001,-2.47908107936455,8.58340091074254));
#46651=CARTESIAN_POINT('Ctrl Pts',(8.,-2.47134253183697,8.56680273025821));
#46652=CARTESIAN_POINT('Ctrl Pts',(8.,-2.46343939564924,8.55026701909029));
#46653=CARTESIAN_POINT('Ctrl Pts',(8.,-2.45734242320857,8.53751033960472));
#46654=CARTESIAN_POINT('Ctrl Pts',(8.,-2.45114811205187,8.52479227107978));
#46655=CARTESIAN_POINT('Ctrl Pts',(8.,-2.44486281855001,8.51212450604301));
#46656=CARTESIAN_POINT('Ctrl Pts',(8.,-2.40201686213332,8.42577014430926));
#46657=CARTESIAN_POINT('Ctrl Pts',(8.00000000000001,-2.35488188271061,8.34161485601582));
#46658=CARTESIAN_POINT('Ctrl Pts',(8.00000000000001,-2.30380034208708,8.25990966013367));
#46659=CARTESIAN_POINT('Ctrl Pts',(8.00000000000001,-2.25170750980348,8.17658689786312));
#46660=CARTESIAN_POINT('Ctrl Pts',(8.,-2.19550998965609,8.09581142569263));
#46661=CARTESIAN_POINT('Ctrl Pts',(8.,-2.1355160195268,8.01785657644985));
#46662=CARTESIAN_POINT('Ctrl Pts',(8.,-2.07504255195389,7.93927867874322));
#46663=CARTESIAN_POINT('Ctrl Pts',(8.,-2.01071124548655,7.86356583221357));
#46664=CARTESIAN_POINT('Ctrl Pts',(8.,-1.94278853690603,7.79101737230827));
#46665=CARTESIAN_POINT('Ctrl Pts',(8.,-1.90599124384239,7.7517140671804));
#46666=CARTESIAN_POINT('Ctrl Pts',(8.,-1.86813908204872,7.71333990439387));
#46667=CARTESIAN_POINT('Ctrl Pts',(8.,-1.82926920156819,7.67594618621562));
#46668=CARTESIAN_POINT('Ctrl Pts',(8.,-1.81677270980972,7.66392427399833));
#46669=CARTESIAN_POINT('Ctrl Pts',(8.00000000000001,-1.80417100132353,7.65200372369101));
#46670=CARTESIAN_POINT('Ctrl Pts',(8.00000000000001,-1.79146523890468,7.64018631111872));
#46671=CARTESIAN_POINT('Ctrl Pts',(8.00000000000001,-1.78112922343272,7.63057295969917));
#46672=CARTESIAN_POINT('Ctrl Pts',(8.,-1.77072739635744,7.62103074875285));
#46673=CARTESIAN_POINT('Ctrl Pts',(8.,-1.76026664533577,7.61156594719198));
#46674=CARTESIAN_POINT('Ctrl Pts',(8.,-1.68459529142931,7.54309912802346));
#46675=CARTESIAN_POINT('Ctrl Pts',(8.,-1.6057511040431,7.47859424872941));
#46676=CARTESIAN_POINT('Ctrl Pts',(8.,-1.52406119076726,7.41833464906689));
#46677=CARTESIAN_POINT('Ctrl Pts',(8.,-1.44227612341757,7.35800485779604));
#46678=CARTESIAN_POINT('Ctrl Pts',(8.,-1.35763812210306,7.30192940135854));
#46679=CARTESIAN_POINT('Ctrl Pts',(8.,-1.2704302700998,7.25041854115382));
#46680=CARTESIAN_POINT('Ctrl Pts',(8.,-1.18495691856711,7.19993219432963));
#46681=CARTESIAN_POINT('Ctrl Pts',(8.,-1.09701426053311,7.15382999685364));
#46682=CARTESIAN_POINT('Ctrl Pts',(8.,-1.00683484042521,7.11244002002564));
#46683=CARTESIAN_POINT('Ctrl Pts',(8.,-0.96920880645403,7.09517066220173));
#46684=CARTESIAN_POINT('Ctrl Pts',(8.,-0.931193028712579,7.07872212712715));
#46685=CARTESIAN_POINT('Ctrl Pts',(8.,-0.892803010639351,7.06312058236777));
#46686=CARTESIAN_POINT('Ctrl Pts',(8.,-0.860663869165804,7.05005936803672));
#46687=CARTESIAN_POINT('Ctrl Pts',(8.,-0.828262419601745,7.03759180517012));
#46688=CARTESIAN_POINT('Ctrl Pts',(8.,-0.795613156383193,7.02571472931219));
#46689=CARTESIAN_POINT('Ctrl Pts',(25.112583302492,-2.51369118594155,10.0007624228313));
#46690=CARTESIAN_POINT('Ctrl Pts',(25.0892658674683,-2.5146904428337,10.3708906137259));
#46691=CARTESIAN_POINT('Ctrl Pts',(25.0659484324445,-2.43811651330385,10.7406256886329));
#46692=CARTESIAN_POINT('Ctrl Pts',(25.0426309974208,-2.28187612815157,11.0729134384505));
#46693=CARTESIAN_POINT('Ctrl Pts',(24.9900302844658,-1.92942073831072,11.8225058584072));
#46694=CARTESIAN_POINT('Ctrl Pts',(24.9374295715108,-1.17155278170321,12.3815335536695));
#46695=CARTESIAN_POINT('Ctrl Pts',(24.8848288585558,-0.351289714219785,
12.4969436943295));
#46696=CARTESIAN_POINT('Ctrl Pts',(24.8322281456008,0.468973353263639,12.6123538349896));
#46697=CARTESIAN_POINT('Ctrl Pts',(24.7796274326458,1.35163153162298,12.2841464210474));
#46698=CARTESIAN_POINT('Ctrl Pts',(24.7270267196908,1.89724190231406,11.6608859500042));
#46699=CARTESIAN_POINT('Ctrl Pts',(24.6744260067358,2.44285227300514,11.0376254789611));
#46700=CARTESIAN_POINT('Ctrl Pts',(24.6218252937808,2.65141483602796,10.1193119508169));
#46701=CARTESIAN_POINT('Ctrl Pts',(24.5692245808258,2.42853259501223,9.32152656027651));
#46702=CARTESIAN_POINT('Ctrl Pts',(24.5166238678708,2.20565035399651,8.52374116973612));
#46703=CARTESIAN_POINT('Ctrl Pts',(24.4640231549158,1.55132330894224,7.84648391679955));
#46704=CARTESIAN_POINT('Ctrl Pts',(24.4114224419608,0.761681514417321,7.59626555006011));
#46705=CARTESIAN_POINT('Ctrl Pts',(24.3588217290058,-0.0279602801076025,
7.34604718332067));
#46706=CARTESIAN_POINT('Ctrl Pts',(24.3062210160508,-0.95291682410319,7.52286770277837));
#46707=CARTESIAN_POINT('Ctrl Pts',(24.2536203030958,-1.59458768801068,8.04670024587429));
#46708=CARTESIAN_POINT('Ctrl Pts',(24.2066079695612,-2.16808646737625,8.51488002612498));
#46709=CARTESIAN_POINT('Ctrl Pts',(24.1595956360266,-2.51529544719306,9.26025447871382));
#46710=CARTESIAN_POINT('Ctrl Pts',(24.112583302492,-2.52041830912221,10.0014523913097));
#46711=CARTESIAN_POINT('Origin',(8.,0.,10.));
#46712=CARTESIAN_POINT('',(8.,0.,20.));
#46713=CARTESIAN_POINT('Origin',(17.,0.,10.));
#46714=CARTESIAN_POINT('Origin',(8.,0.,10.));
#46715=CARTESIAN_POINT('',(8.,0.,20.));
#46716=CARTESIAN_POINT('Origin',(0.,0.,20.));
#46717=CARTESIAN_POINT('',(8.,9.79717439317883E-16,-5.));
#46718=CARTESIAN_POINT('Origin',(0.,0.,-5.));
#46719=CARTESIAN_POINT('',(8.,9.79717439317883E-16,20.));
#46720=CARTESIAN_POINT('',(8.,9.79717439317883E-16,40.));
#46721=CARTESIAN_POINT('',(8.,9.79717439317883E-16,20.));
#46722=CARTESIAN_POINT('Origin',(0.,0.,40.));
#46723=CARTESIAN_POINT('Origin',(0.,0.,40.));
#46724=CARTESIAN_POINT('Origin',(0.,0.,220.));
#46725=CARTESIAN_POINT('',(-12.,-1.46957615897682E-15,265.));
#46726=CARTESIAN_POINT('Origin',(0.,0.,265.));
#46727=CARTESIAN_POINT('',(-12.,-1.46957615897682E-15,220.));
#46728=CARTESIAN_POINT('Origin',(0.,0.,265.));
#46729=CARTESIAN_POINT('Origin',(0.,0.,41.));
#46730=CARTESIAN_POINT('',(-26.,-3.18408167778312E-15,41.));
#46731=CARTESIAN_POINT('Origin',(0.,0.,41.));
#46732=CARTESIAN_POINT('',(-20.,-2.44929359829471E-15,41.));
#46733=CARTESIAN_POINT('Origin',(0.,0.,41.));
#46734=CARTESIAN_POINT('Origin',(0.,0.,37.));
#46735=CARTESIAN_POINT('',(-26.,-3.18408167778312E-15,37.));
#46736=CARTESIAN_POINT('Origin',(0.,0.,37.));
#46737=CARTESIAN_POINT('',(-20.,2.44929359829471E-15,37.));
#46738=CARTESIAN_POINT('Origin',(0.,0.,37.));
#46739=CARTESIAN_POINT('Origin',(0.,0.,37.));
#46740=CARTESIAN_POINT('',(-26.,-3.18408167778312E-15,37.));
#46741=CARTESIAN_POINT('Origin',(0.,0.,20.));
#46742=CARTESIAN_POINT('',(-20.,-2.44929359829471E-15,20.));
#46743=CARTESIAN_POINT('',(-20.,-2.44929359829471E-15,20.));
#46744=CARTESIAN_POINT('Origin',(0.,0.,20.));
#46745=CARTESIAN_POINT('Origin',(0.,0.,20.));
#46746=CARTESIAN_POINT('',(-26.,-3.18408167778312E-15,20.));
#46747=CARTESIAN_POINT('Origin',(0.,0.,20.));
#46748=CARTESIAN_POINT('Origin',(0.,0.,0.));
#46749=CARTESIAN_POINT('',(-26.,-3.18408167778312E-15,-5.));
#46750=CARTESIAN_POINT('',(-26.,-3.18408167778312E-15,0.));
#46751=CARTESIAN_POINT('Origin',(0.,0.,-5.));
#46752=CARTESIAN_POINT('Origin',(0.,0.,-5.));
#46753=CARTESIAN_POINT('Origin',(0.,0.,20.));
#46754=CARTESIAN_POINT('',(-20.,-2.44929359829471E-15,20.));
#63862=UNCERTAINTY_MEASURE_WITH_UNIT(LENGTH_MEASURE(0.01),#63899,
'DISTANCE_ACCURACY_VALUE',
'Maximum model space distance between geometric entities at asserted c
onnectivities');
#63878=UNCERTAINTY_MEASURE_WITH_UNIT(LENGTH_MEASURE(0.01),#63899,
'DISTANCE_ACCURACY_VALUE',
'Maximum model space distance between geometric entities at asserted c
onnectivities');
#63882=(
GEOMETRIC_REPRESENTATION_CONTEXT(3)
GLOBAL_UNCERTAINTY_ASSIGNED_CONTEXT((#63862))
GLOBAL_UNIT_ASSIGNED_CONTEXT((#63899,#63901,#63902))
REPRESENTATION_CONTEXT('','3D')
);
#63898=(
GEOMETRIC_REPRESENTATION_CONTEXT(3)
GLOBAL_UNCERTAINTY_ASSIGNED_CONTEXT((#63878))
GLOBAL_UNIT_ASSIGNED_CONTEXT((#63899,#63901,#63902))
REPRESENTATION_CONTEXT('','3D')
);
#63899=(
LENGTH_UNIT()
NAMED_UNIT(*)
SI_UNIT(.MILLI.,.METRE.)
);
#63901=(
NAMED_UNIT(*)
PLANE_ANGLE_UNIT()
SI_UNIT($,.RADIAN.)
);
#63902=(
NAMED_UNIT(*)
SI_UNIT($,.STERADIAN.)
SOLID_ANGLE_UNIT()
);
#63906=SHAPE_DEFINITION_REPRESENTATION(#63925,#63997);
#63925=PRODUCT_DEFINITION_SHAPE('',$,#64017);
#63997=SHAPE_REPRESENTATION('',(#16184),#63882);
#64013=PRODUCT_DEFINITION_CONTEXT('part definition',#64072,'design');
#64017=PRODUCT_DEFINITION('Spindle','Spindle',#64036,#64013);
#64036=PRODUCT_DEFINITION_FORMATION('',$,#64077);
#64072=APPLICATION_CONTEXT(
'Core Data for Automotive Mechanical Design Process');
#64073=PRODUCT_CONTEXT('part definition',#64072,'mechanical');
#64077=PRODUCT('Spindle','Spindle',$,(#64073));
#64096=PRESENTATION_STYLE_ASSIGNMENT((#64109));
#64109=SURFACE_STYLE_USAGE(.BOTH.,#64122);
#64122=SURFACE_SIDE_STYLE('',(#64135));
#64135=SURFACE_STYLE_FILL_AREA(#64148);
#64148=FILL_AREA_STYLE('Spindle gray',(#64161));
#64161=FILL_AREA_STYLE_COLOUR('Spindle gray',#64174);
#64174=COLOUR_RGB('Spindle gray',0.576470588235294,0.615686274509804,0.666666666666667);
ENDSEC;
END-ISO-10303-21;
